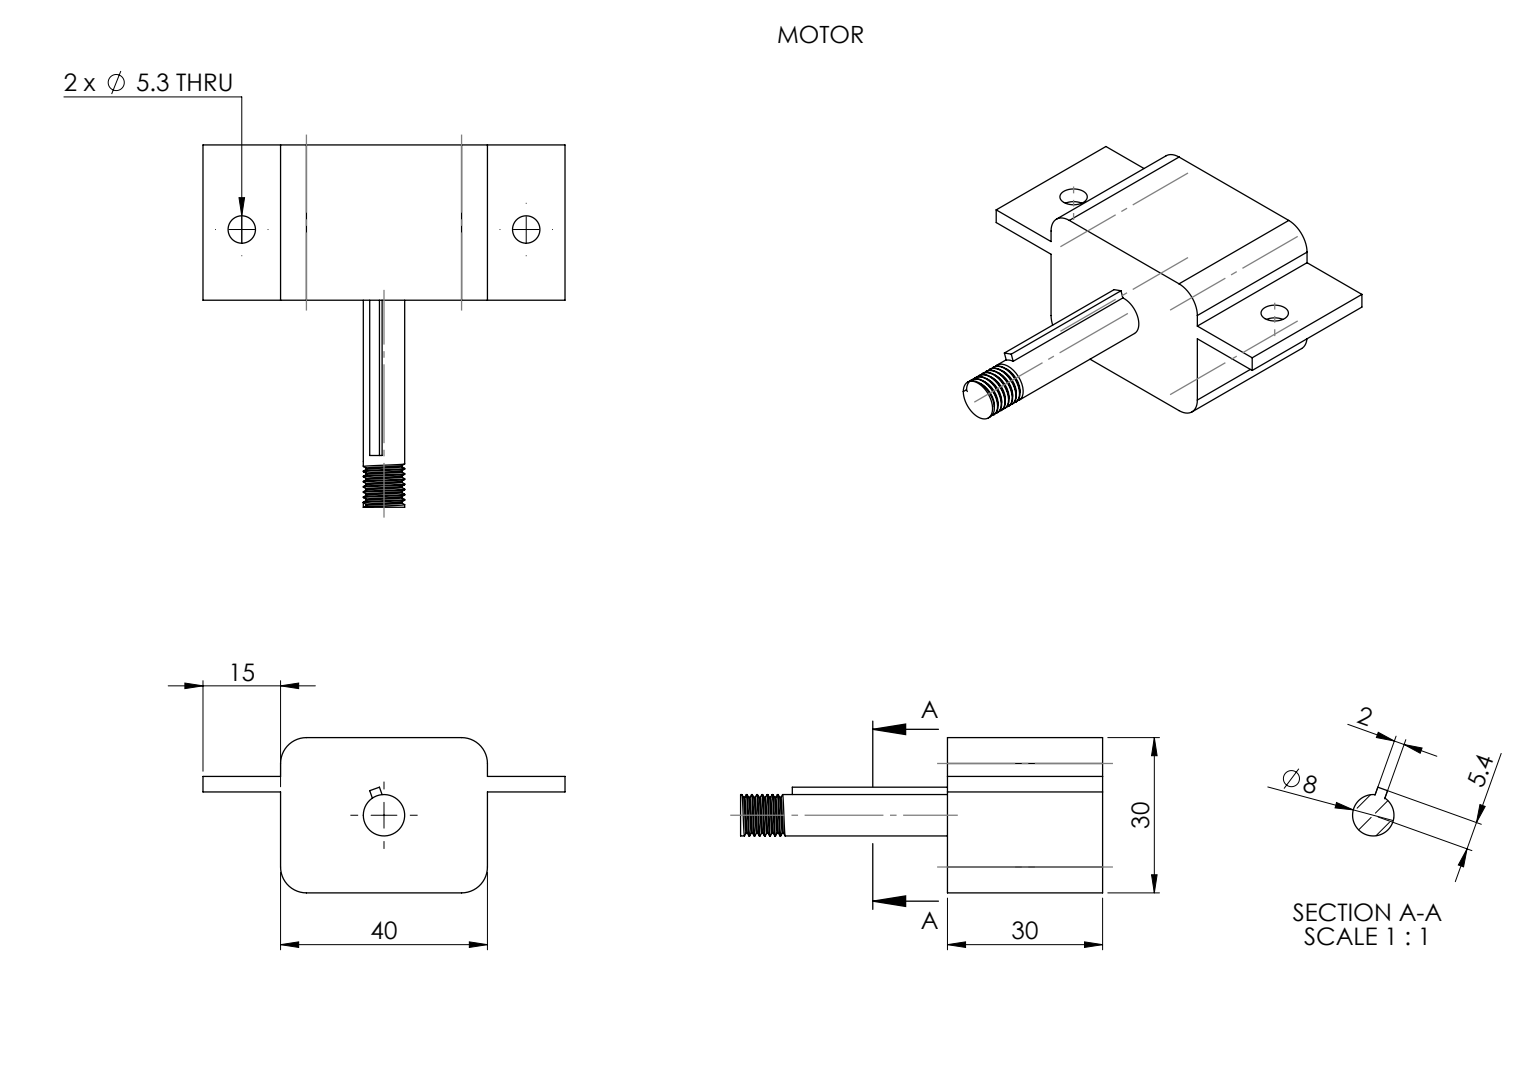
ISO-10303-21;
HEADER;
FILE_DESCRIPTION (('STEP AP214'),
    '1' );
FILE_NAME ('motor.step',
    '2026-10-08T13:46:47',
    ( '' ),
    ( '' ),
    'SwSTEP 2.0',
    'SolidWorks 2026',
    '' );
FILE_SCHEMA (( 'AUTOMOTIVE_DESIGN' ));
ENDSEC;

DATA;
#1=CARTESIAN_POINT ( 'NONE',  ( -3.999999999999999112, 1.656854249492380804, 17.93750000000000711 ) ) ;
#3=VECTOR ( 'NONE', #11246, 1000.000000000000000 ) ;
#10=DIRECTION ( 'NONE',  ( -0.000000000000000000, -0.000000000000000000, -1.000000000000000000 ) ) ;
#11=CARTESIAN_POINT ( 'NONE',  ( 1.432654583217641164, 3.458734125000000326, 19.12500000136560629 ) ) ;
#16=CARTESIAN_POINT ( 'NONE',  ( 2.445694354108821855, -2.445694354108820079, 11.81250000136560629 ) ) ;
#34=CARTESIAN_POINT ( 'NONE',  ( -1.432654583217639832, -3.458734125000000326, 12.87500000136560629 ) ) ;
#40=CARTESIAN_POINT ( 'NONE',  ( -3.999999999999999112, 0.000000000000000000, 16.12500000273119838 ) ) ;
#41=CARTESIAN_POINT ( 'NONE',  ( -20.00000000000000711, 9.999999999999964473, -19.99999999999999645 ) ) ;
#44=CYLINDRICAL_SURFACE ( 'NONE', #19665, 4.000000000000000000 ) ;
#50=ORIENTED_EDGE ( 'NONE', *, *, #19475, .F. ) ;
#51=CARTESIAN_POINT ( 'NONE',  ( -3.999999999999999112, 1.656854249492380804, 17.93750000000000711 ) ) ;
#54=ORIENTED_EDGE ( 'NONE', *, *, #9397, .T. ) ;
#64=CARTESIAN_POINT ( 'NONE',  ( -2.445694354108819191, 2.445694354108820523, 10.31250000136560629 ) ) ;
#82=ADVANCED_FACE ( 'NONE', ( #16139 ), #13987, .T. ) ;
#87=CARTESIAN_POINT ( 'NONE',  ( -2.828427124746189403, 2.828427124746190291, 10.87500000000001066 ) ) ;
#108=CARTESIAN_POINT ( 'NONE',  ( 4.000000000000000888, 4.898587196589412829E-16, 18.50000000000001066 ) ) ;
#110=EDGE_CURVE ( 'NONE', #1631, #9768, #19532, .T. ) ;
#115=ORIENTED_EDGE ( 'NONE', *, *, #19552, .T. ) ;
#121=CARTESIAN_POINT ( 'NONE',  ( 1.025207404391860050E-15, 3.458734125000000326, 19.18750000136560629 ) ) ;
#124=CARTESIAN_POINT ( 'NONE',  ( -3.999999999999999112, 0.000000000000000000, 13.00000000000001066 ) ) ;
#125=CARTESIAN_POINT ( 'NONE',  ( 1.432654583217641164, 3.458734125000000326, 12.12500000136560629 ) ) ;
#139=CARTESIAN_POINT ( 'NONE',  ( 1.025207404391860050E-15, 3.458734125000000770, 19.43750000136560629 ) ) ;
#149=DIRECTION ( 'NONE',  ( -0.000000000000000000, 1.000000000000000000, -0.000000000000000000 ) ) ;
#152=CARTESIAN_POINT ( 'NONE',  ( 2.828427124746191179, 2.828427124746190291, 16.75000000273119838 ) ) ;
#158=VERTEX_POINT ( 'NONE', #14232 ) ;
#164=CARTESIAN_POINT ( 'NONE',  ( 1.971781867644420635E-15, -4.000000000000000000, 16.25000000000001066 ) ) ;
#171=ADVANCED_FACE ( 'NONE', ( #19699 ), #12685, .T. ) ;
#180=CARTESIAN_POINT ( 'NONE',  ( 3.458734125000002546, -1.432654583217639610, 15.12500000136560807 ) ) ;
#183=CARTESIAN_POINT ( 'NONE',  ( 9.920644283265380691E-16, 4.000000000000000000, 16.75000000000001066 ) ) ;
#185=CARTESIAN_POINT ( 'NONE',  ( 1.656854249492381470, 4.000000000000000000, 11.81250000273119660 ) ) ;
#188=EDGE_LOOP ( 'NONE', ( #20058, #4346, #18980, #11606 ) ) ;
#189=ORIENTED_EDGE ( 'NONE', *, *, #1029, .F. ) ;
#190=LINE ( 'NONE', #7521, #665 ) ;
#194=CARTESIAN_POINT ( 'NONE',  ( -2.828427124746188515, -2.828427124746190735, 18.12500000000001066 ) ) ;
#202=CARTESIAN_POINT ( 'NONE',  ( 9.920644283265380691E-16, 4.000000000000000000, 15.87500000273119660 ) ) ;
#207=CARTESIAN_POINT ( 'NONE',  ( -2.762848947613220307, 4.746226468750993632, -19.99999999999999645 ) ) ;
#225=CARTESIAN_POINT ( 'NONE',  ( 4.000000000000000888, 4.898587196589412829E-16, 15.50000000000001066 ) ) ;
#234=CARTESIAN_POINT ( 'NONE',  ( 1.432654583217643163, -3.458734124999999437, 15.75000000136560629 ) ) ;
#238=CARTESIAN_POINT ( 'NONE',  ( -3.458734124999998993, 1.432654583217640276, 12.37500000136560629 ) ) ;
#251=CARTESIAN_POINT ( 'NONE',  ( 3.458734125000001658, 1.432654583217640498, 17.25000000136560629 ) ) ;
#257=CARTESIAN_POINT ( 'NONE',  ( 3.458734125000001658, 1.432654583217640498, 13.25000000136560274 ) ) ;
#263=CARTESIAN_POINT ( 'NONE',  ( -1.432654583217638944, 3.458734125000000326, 12.25000000136560629 ) ) ;
#264=CARTESIAN_POINT ( 'NONE',  ( 4.000000000000001776, -1.656854249492379694, 16.56250000273119838 ) ) ;
#265=DIRECTION ( 'NONE',  ( -1.000000000000000000, 0.000000000000000000, 0.000000000000000000 ) ) ;
#272=ORIENTED_EDGE ( 'NONE', *, *, #1937, .F. ) ;
#277=EDGE_LOOP ( 'NONE', ( #17839, #20951 ) ) ;
#278=CARTESIAN_POINT ( 'NONE',  ( 4.000000000000001776, -1.656854249492379694, 13.43750000000001243 ) ) ;
#285=DIRECTION ( 'NONE',  ( -0.000000000000000000, -0.000000000000000000, -1.000000000000000000 ) ) ;
#294=CARTESIAN_POINT ( 'NONE',  ( 1.432654583217641386, 3.458734125000000770, 13.37500000136560452 ) ) ;
#303=CARTESIAN_POINT ( 'NONE',  ( -2.247776618166699603, 3.308700692843501656, 21.31370849898476649 ) ) ;
#315=VERTEX_POINT ( 'NONE', #10985 ) ;
#323=CARTESIAN_POINT ( 'NONE',  ( 1.656854249492384135, -3.999999999999999112, 17.43750000273119483 ) ) ;
#332=ORIENTED_EDGE ( 'NONE', *, *, #12450, .T. ) ;
#343=CARTESIAN_POINT ( 'NONE',  ( 1.656854249492384135, -3.999999999999999112, 16.43750000273119838 ) ) ;
#350=CARTESIAN_POINT ( 'NONE',  ( -2.828427124746189403, 2.828427124746190291, 12.87500000000001066 ) ) ;
#355=AXIS2_PLACEMENT_3D ( 'NONE', #12842, #20101, #14526 ) ;
#361=CARTESIAN_POINT ( 'NONE',  ( 1.025207404391860050E-15, 3.458734125000000326, 17.18750000136560274 ) ) ;
#367=CARTESIAN_POINT ( 'NONE',  ( -2.445694354108819191, 2.445694354108820523, 15.31250000136560452 ) ) ;
#381=CARTESIAN_POINT ( 'NONE',  ( 1.432654583217641386, 3.458734125000000770, 15.37500000136560807 ) ) ;
#383=VECTOR ( 'NONE', #917, 1000.000000000000000 ) ;
#385=AXIS2_PLACEMENT_3D ( 'NONE', #6028, #512, #265 ) ;
#389=CARTESIAN_POINT ( 'NONE',  ( 2.445694354108822299, -2.445694354108820079, 12.06250000136560629 ) ) ;
#395=CARTESIAN_POINT ( 'NONE',  ( -3.999999999999999112, 0.000000000000000000, 17.12500000273119838 ) ) ;
#396=EDGE_CURVE ( 'NONE', #2255, #17303, #7746, .T. ) ;
#409=CARTESIAN_POINT ( 'NONE',  ( 4.000000000000001776, -1.656854249492379694, 12.43750000000001066 ) ) ;
#423=CARTESIAN_POINT ( 'NONE',  ( -1.432654583217639832, -3.458734125000000326, 14.87500000136560807 ) ) ;
#427=CARTESIAN_POINT ( 'NONE',  ( 2.828427124746191179, 2.828427124746190291, 16.62500000000001066 ) ) ;
#429=CARTESIAN_POINT ( 'NONE',  ( -2.828427124746188515, -2.828427124746190735, 14.12500000000001066 ) ) ;
#447=CARTESIAN_POINT ( 'NONE',  ( -1.656854249492380138, -3.999999999999999112, 13.31250000273119660 ) ) ;
#455=EDGE_CURVE ( 'NONE', #7307, #20911, #18012, .T. ) ;
#471=CARTESIAN_POINT ( 'NONE',  ( -2.828427124746189403, 2.828427124746190291, 13.87500000000001066 ) ) ;
#482=CARTESIAN_POINT ( 'NONE',  ( 3.458734125000001214, 1.432654583217640498, 14.00000000136560629 ) ) ;
#488=CARTESIAN_POINT ( 'NONE',  ( 2.445694354108821855, -2.445694354108820079, 13.81250000136560629 ) ) ;
#491=CARTESIAN_POINT ( 'NONE',  ( -2.828427124746189403, 2.828427124746190291, 16.00000000273119838 ) ) ;
#500=CARTESIAN_POINT ( 'NONE',  ( 1.432654583217643163, -3.458734124999999882, 15.00000000136560629 ) ) ;
#510=CARTESIAN_POINT ( 'NONE',  ( -2.445694354108819191, 2.445694354108820523, 10.31250000136560629 ) ) ;
#511=CARTESIAN_POINT ( 'NONE',  ( 1.971781867644420635E-15, -4.000000000000000000, 14.37500000273119660 ) ) ;
#512=DIRECTION ( 'NONE',  ( -1.224646799147353207E-16, 0.000000000000000000, -1.000000000000000000 ) ) ;
#514=ORIENTED_EDGE ( 'NONE', *, *, #14781, .F. ) ;
#523=CARTESIAN_POINT ( 'NONE',  ( 1.656854249492384135, -3.999999999999999112, 12.31250000000001243 ) ) ;
#536=CARTESIAN_POINT ( 'NONE',  ( -1.432654583217639166, 3.458734125000000770, 16.50000000136560629 ) ) ;
#554=CARTESIAN_POINT ( 'NONE',  ( 4.000000000000000888, 4.898587196589412829E-16, 19.50000000000001066 ) ) ;
#558=CARTESIAN_POINT ( 'NONE',  ( 2.828427124746191179, 2.828427124746190291, 13.75000000273119483 ) ) ;
#562=CARTESIAN_POINT ( 'NONE',  ( 3.458734125000001214, 1.432654583217640498, 19.00000000136560629 ) ) ;
#582=CARTESIAN_POINT ( 'NONE',  ( 4.000000000000000888, 4.898587196589412829E-16, 13.50000000000001066 ) ) ;
#587=CARTESIAN_POINT ( 'NONE',  ( 27.50000000000000000, 4.500000000000001776, -36.31025403784445871 ) ) ;
#590=VECTOR ( 'NONE', #2193, 1000.000000000000000 ) ;
#594=CARTESIAN_POINT ( 'NONE',  ( 1.432654583217641164, 3.458734125000000326, 13.12500000136560274 ) ) ;
#598=CARTESIAN_POINT ( 'NONE',  ( -3.999999999999999112, 1.656854249492380582, 12.93750000000001066 ) ) ;
#613=ORIENTED_EDGE ( 'NONE', *, *, #10738, .T. ) ;
#614=CARTESIAN_POINT ( 'NONE',  ( 1.025207404391860050E-15, 3.458734125000000770, 18.43750000136560629 ) ) ;
#625=CARTESIAN_POINT ( 'NONE',  ( 2.445694354108821855, -2.445694354108820079, 10.81250000136560452 ) ) ;
#626=CARTESIAN_POINT ( 'NONE',  ( 2.828427124746191179, 2.828427124746190291, 11.75000000273119660 ) ) ;
#629=ORIENTED_EDGE ( 'NONE', *, *, #21485, .F. ) ;
#634=CARTESIAN_POINT ( 'NONE',  ( 2.828427124746192067, -2.828427124746189847, 11.37500000000001066 ) ) ;
#636=EDGE_CURVE ( 'NONE', #21119, #17601, #4711, .T. ) ;
#644=CARTESIAN_POINT ( 'NONE',  ( -3.458734124999998105, -1.432654583217642497, 18.75000000136560985 ) ) ;
#645=CARTESIAN_POINT ( 'NONE',  ( 4.000000000000000888, 4.898587196589412829E-16, 11.50000000000001066 ) ) ;
#651=CARTESIAN_POINT ( 'NONE',  ( -1.432654583217639166, 3.458734125000000770, 14.50000000136560629 ) ) ;
#652=DIRECTION ( 'NONE',  ( -1.224646799147353207E-16, 0.000000000000000000, -1.000000000000000000 ) ) ;
#659=ORIENTED_EDGE ( 'NONE', *, *, #9537, .F. ) ;
#662=CARTESIAN_POINT ( 'NONE',  ( 4.000000000000000888, 4.898587196589412829E-16, 21.31370849898476649 ) ) ;
#665=VECTOR ( 'NONE', #22333, 1000.000000000000000 ) ;
#673=( BOUNDED_CURVE ( )  B_SPLINE_CURVE ( 2, ( #7283, #9203, #16490, #14354, #12440, #10774, #7037, #12692, #3655 ),
 .UNSPECIFIED., .F., .F. ) 
 B_SPLINE_CURVE_WITH_KNOTS ( ( 3, 2, 2, 2, 3 ),
 ( 0.05000000000000000278, 0.06250000000000000000, 0.07499999999999999722, 0.08749999999999999445, 0.1000000000000000056 ),
 .UNSPECIFIED. ) 
 CURVE ( )  GEOMETRIC_REPRESENTATION_ITEM ( )  RATIONAL_B_SPLINE_CURVE ( ( 1.000000000000000000, 0.9238795325112867385, 1.000000000000000000, 0.9238795325112867385, 1.000000000000000000, 0.9238795325112867385, 1.000000000000000000, 0.9238795325112867385, 1.000000000000000000 ) ) 
 REPRESENTATION_ITEM ( '' )  );
#676=CARTESIAN_POINT ( 'NONE',  ( -2.445694354108818303, -2.445694354108820523, 18.56250000136560629 ) ) ;
#694=FACE_OUTER_BOUND ( 'NONE', #17938, .T. ) ;
#698=CARTESIAN_POINT ( 'NONE',  ( 4.000000000000000888, 1.656854249492381248, 16.56250000000001066 ) ) ;
#706=ADVANCED_FACE ( 'NONE', ( #20086 ), #19862, .T. ) ;
#709=DIRECTION ( 'NONE',  ( -0.000000000000000000, -0.000000000000000000, -1.000000000000000000 ) ) ;
#712=CARTESIAN_POINT ( 'NONE',  ( 2.445694354108821855, -2.445694354108820079, 11.81250000136560629 ) ) ;
#724=ORIENTED_EDGE ( 'NONE', *, *, #7005, .T. ) ;
#725=CARTESIAN_POINT ( 'NONE',  ( -3.999999999999999112, 0.000000000000000000, 16.12500000273119838 ) ) ;
#736=CARTESIAN_POINT ( 'NONE',  ( -2.445694354108818303, -2.445694354108820967, 16.81250000136560629 ) ) ;
#749=CARTESIAN_POINT ( 'NONE',  ( -3.999999999999998224, -1.656854249492383246, 13.18750000273119660 ) ) ;
#756=CARTESIAN_POINT ( 'NONE',  ( -2.828427124746189403, 2.828427124746190291, 17.00000000273119838 ) ) ;
#764=CARTESIAN_POINT ( 'NONE',  ( 1.656854249492384135, -3.999999999999999112, 14.31250000000001066 ) ) ;
#767=ORIENTED_EDGE ( 'NONE', *, *, #14910, .F. ) ;
#772=CARTESIAN_POINT ( 'NONE',  ( 2.445694354108822299, -2.445694354108820079, 18.06250000136560274 ) ) ;
#774=VECTOR ( 'NONE', #12841, 1000.000000000000000 ) ;
#780=CARTESIAN_POINT ( 'NONE',  ( 3.458734125000001658, 1.432654583217640498, 12.25000000136560452 ) ) ;
#781=ADVANCED_FACE ( 'NONE', ( #23460 ), #8880, .F. ) ;
#784=EDGE_CURVE ( 'NONE', #20532, #22990, #16520, .T. ) ;
#786=LINE ( 'NONE', #11832, #6692 ) ;
#795=EDGE_LOOP ( 'NONE', ( #3413, #2892, #4216, #3819, #4414, #8132, #9324, #7494, #20640, #8419, #9699, #7965, #332, #11494, #6870, #4116, #6329, #19356, #12885, #18929, #9383, #2214 ) ) ;
#800=ORIENTED_EDGE ( 'NONE', *, *, #8131, .T. ) ;
#801=FACE_OUTER_BOUND ( 'NONE', #1222, .T. ) ;
#803=CARTESIAN_POINT ( 'NONE',  ( -1.432654583217638944, 3.458734125000000326, 18.25000000136560629 ) ) ;
#819=ADVANCED_FACE ( 'NONE', ( #14739 ), #5612, .T. ) ;
#821=CARTESIAN_POINT ( 'NONE',  ( 4.000000000000000888, 1.656854249492381248, 12.56250000000001243 ) ) ;
#823=CARTESIAN_POINT ( 'NONE',  ( 4.000000000000000888, 4.898587196589412829E-16, 19.50000000000001066 ) ) ;
#824=( BOUNDED_CURVE ( )  B_SPLINE_CURVE ( 2, ( #13954, #15639, #17660, #1221, #6398, #22911, #21329, #10248, #6525 ),
 .UNSPECIFIED., .F., .F. ) 
 B_SPLINE_CURVE_WITH_KNOTS ( ( 3, 2, 2, 2, 3 ),
 ( 0.000000000000000000, 0.01250000000000000243, 0.02500000000000000486, 0.03749999999999999861, 0.05000000000000000971 ),
 .UNSPECIFIED. ) 
 CURVE ( )  GEOMETRIC_REPRESENTATION_ITEM ( )  RATIONAL_B_SPLINE_CURVE ( ( 1.000000000000000000, 0.9238795325112867385, 1.000000000000000000, 0.9238795325112867385, 1.000000000000000000, 0.9238795325112867385, 1.000000000000000000, 0.9238795325112867385, 1.000000000000000000 ) ) 
 REPRESENTATION_ITEM ( '' )  );
#830=CARTESIAN_POINT ( 'NONE',  ( 1.872352939448454495E-15, -3.458734125000000326, 11.68750000136560629 ) ) ;
#832=CYLINDRICAL_SURFACE ( 'NONE', #7334, 4.999999999999997335 ) ;
#836=CARTESIAN_POINT ( 'NONE',  ( 1.872352939448454495E-15, -3.458734125000000326, 10.68750000136560452 ) ) ;
#839=VERTEX_POINT ( 'NONE', #9344 ) ;
#848=CARTESIAN_POINT ( 'NONE',  ( -2.445694354108818303, -2.445694354108820967, 13.81250000136560629 ) ) ;
#856=PLANE ( 'NONE',  #19991 ) ;
#859=CARTESIAN_POINT ( 'NONE',  ( -3.999999999999999112, 0.000000000000000000, 10.12500000273119660 ) ) ;
#860=FACE_OUTER_BOUND ( 'NONE', #12699, .T. ) ;
#863=EDGE_LOOP ( 'NONE', ( #11160, #1862, #19901, #14870 ) ) ;
#867=ORIENTED_EDGE ( 'NONE', *, *, #22089, .F. ) ;
#878=DIRECTION ( 'NONE',  ( -0.000000000000000000, -0.000000000000000000, -1.000000000000000000 ) ) ;
#891=DIRECTION ( 'NONE',  ( -1.224646799147353207E-16, 0.000000000000000000, -1.000000000000000000 ) ) ;
#893=CARTESIAN_POINT ( 'NONE',  ( -3.999999999999999112, 0.000000000000000000, 14.00000000000001066 ) ) ;
#913=CARTESIAN_POINT ( 'NONE',  ( 1.872352939448454495E-15, -3.458734125000000326, 18.68750000136560629 ) ) ;
#916=ORIENTED_EDGE ( 'NONE', *, *, #11727, .T. ) ;
#917=DIRECTION ( 'NONE',  ( -0.000000000000000000, -0.000000000000000000, -1.000000000000000000 ) ) ;
#927=CYLINDRICAL_SURFACE ( 'NONE', #10317, 4.000000000000000000 ) ;
#940=CARTESIAN_POINT ( 'NONE',  ( -3.458734124999998993, 1.432654583217640276, 14.37500000136560452 ) ) ;
#950=CARTESIAN_POINT ( 'NONE',  ( 1.025207404391860050E-15, 3.458734125000000326, 10.18750000136560629 ) ) ;
#953=DIRECTION ( 'NONE',  ( 0.000000000000000000, 0.000000000000000000, 1.000000000000000000 ) ) ;
#961=CARTESIAN_POINT ( 'NONE',  ( 3.458734125000001658, 4.235727675282972223E-16, 13.18750000136560452 ) ) ;
#976=CARTESIAN_POINT ( 'NONE',  ( 1.656854249492384135, -3.999999999999999112, 13.43750000273119838 ) ) ;
#977=DIRECTION ( 'NONE',  ( 0.3373062947069098150, -0.9413949561959078505, 0.000000000000000000 ) ) ;
#988=DIRECTION ( 'NONE',  ( 1.000000000000000000, 0.000000000000000000, 0.000000000000000000 ) ) ;
#996=DIRECTION ( 'NONE',  ( -0.000000000000000000, -0.000000000000000000, -1.000000000000000000 ) ) ;
#998=CARTESIAN_POINT ( 'NONE',  ( 2.828427124746191179, 2.828427124746190291, 15.75000000273119660 ) ) ;
#1006=CARTESIAN_POINT ( 'NONE',  ( 1.432654583217643163, -3.458734124999999882, 13.00000000136560629 ) ) ;
#1012=CARTESIAN_POINT ( 'NONE',  ( 4.000000000000000888, 4.898587196589412829E-16, 15.62500000273119660 ) ) ;
#1013=PRESENTATION_STYLE_ASSIGNMENT (( #17448 ) ) ;
#1029=EDGE_CURVE ( 'NONE', #4019, #13418, #23047, .T. ) ;
#1031=CARTESIAN_POINT ( 'NONE',  ( -2.445694354108819191, 2.445694354108820523, 19.31250000136560629 ) ) ;
#1049=CARTESIAN_POINT ( 'NONE',  ( 2.828427124746191179, 2.828427124746190291, 17.62500000000001066 ) ) ;
#1053=CARTESIAN_POINT ( 'NONE',  ( -3.999999999999999112, 0.000000000000000000, 12.00000000000001066 ) ) ;
#1060=CARTESIAN_POINT ( 'NONE',  ( -1.432654583217639166, 3.458734125000000770, 18.50000000136560629 ) ) ;
#1065=CARTESIAN_POINT ( 'NONE',  ( 1.656854249492381470, 4.000000000000000000, 15.68750000000001066 ) ) ;
#1080=CARTESIAN_POINT ( 'NONE',  ( -3.458734124999999437, 1.432654583217640498, 11.62500000136560452 ) ) ;
#1092=CARTESIAN_POINT ( 'NONE',  ( 4.000000000000000888, 4.898587196589412829E-16, 12.62500000273119660 ) ) ;
#1112=CARTESIAN_POINT ( 'NONE',  ( -3.458734124999998105, -1.432654583217642497, 17.75000000136560274 ) ) ;
#1113=CARTESIAN_POINT ( 'NONE',  ( -2.828427124746188515, -2.828427124746190735, 14.25000000273119660 ) ) ;
#1114=VECTOR ( 'NONE', #23199, 1000.000000000000000 ) ;
#1127=CARTESIAN_POINT ( 'NONE',  ( 1.971781867644420635E-15, -4.000000000000000000, 15.37500000273119660 ) ) ;
#1128=( NAMED_UNIT ( * ) PLANE_ANGLE_UNIT ( ) SI_UNIT ( $, .RADIAN. ) );
#1132=VERTEX_POINT ( 'NONE', #18132 ) ;
#1136=FACE_OUTER_BOUND ( 'NONE', #3145, .T. ) ;
#1138=UNCERTAINTY_MEASURE_WITH_UNIT (LENGTH_MEASURE( 1.000000000000000082E-05 ), #18255, 'distance_accuracy_value', 'NONE');
#1146=DIRECTION ( 'NONE',  ( -1.000000000000000000, 0.000000000000000000, 0.000000000000000000 ) ) ;
#1150=CARTESIAN_POINT ( 'NONE',  ( 2.445694354108821411, 2.445694354108820523, 16.06250000136560629 ) ) ;
#1166=ORIENTED_EDGE ( 'NONE', *, *, #12523, .F. ) ;
#1167=CARTESIAN_POINT ( 'NONE',  ( -3.999999999999999112, 0.000000000000000000, 20.00000000000001066 ) ) ;
#1170=CARTESIAN_POINT ( 'NONE',  ( -1.656854249492380138, -3.999999999999999112, 19.18750000000001066 ) ) ;
#1176=EDGE_CURVE ( 'NONE', #158, #17446, #12413, .T. ) ;
#1178=CARTESIAN_POINT ( 'NONE',  ( -15.00000000000001066, 10.00000000000000000, -49.99999999999999289 ) ) ;
#1181=CARTESIAN_POINT ( 'NONE',  ( 2.445694354108821855, -2.445694354108820079, 10.81250000136560452 ) ) ;
#1196=ORIENTED_EDGE ( 'NONE', *, *, #6597, .F. ) ;
#1197=CARTESIAN_POINT ( 'NONE',  ( -1.432654583217639166, 3.458734125000000770, 13.50000000136560452 ) ) ;
#1209=CARTESIAN_POINT ( 'NONE',  ( -3.458734124999998993, -1.432654583217642497, 18.50000000136560629 ) ) ;
#1221=CARTESIAN_POINT ( 'NONE',  ( -1.656854249492379472, 4.000000000000000000, 19.81250000000001776 ) ) ;
#1222=EDGE_LOOP ( 'NONE', ( #3301, #17935, #17506, #2754 ) ) ;
#1227=CARTESIAN_POINT ( 'NONE',  ( 3.458734125000001658, 1.432654583217640498, 14.25000000136560452 ) ) ;
#1228=CARTESIAN_POINT ( 'NONE',  ( -1.656854249492379250, 4.000000000000000000, 14.93750000273119660 ) ) ;
#1233=CARTESIAN_POINT ( 'NONE',  ( -3.458734124999999437, 1.432654583217640498, 11.62500000136560452 ) ) ;
#1236=EDGE_CURVE ( 'NONE', #10607, #14136, #2968, .T. ) ;
#1242=SURFACE_STYLE_FILL_AREA ( #17329 ) ;
#1256=DIRECTION ( 'NONE',  ( 1.224646799147353207E-16, -0.000000000000000000, 1.000000000000000000 ) ) ;
#1259=CARTESIAN_POINT ( 'NONE',  ( -1.432654583217638944, 3.458734125000000326, 14.25000000136560452 ) ) ;
#1270=CARTESIAN_POINT ( 'NONE',  ( 4.000000000000000888, 4.898587196589412829E-16, 13.62500000273119660 ) ) ;
#1280=DIRECTION ( 'NONE',  ( -1.224646799147353207E-16, 0.000000000000000000, -1.000000000000000000 ) ) ;
#1281=DIRECTION ( 'NONE',  ( 1.224646799147353207E-16, -0.000000000000000000, 1.000000000000000000 ) ) ;
#1288=CARTESIAN_POINT ( 'NONE',  ( 3.458734125000001214, 4.235727675282971730E-16, 10.93750000136560452 ) ) ;
#1293=DIRECTION ( 'NONE',  ( -0.000000000000000000, -1.000000000000000000, 0.000000000000000000 ) ) ;
#1309=CARTESIAN_POINT ( 'NONE',  ( 1.872352939448454495E-15, -3.458734125000000770, 11.93750000136560629 ) ) ;
#1318=DIRECTION ( 'NONE',  ( -0.000000000000000000, -0.000000000000000000, -1.000000000000000000 ) ) ;
#1323=CARTESIAN_POINT ( 'NONE',  ( 3.458734125000002102, -1.432654583217639610, 17.87500000136560274 ) ) ;
#1332=DIRECTION ( 'NONE',  ( -0.000000000000000000, -1.000000000000000000, 0.000000000000000000 ) ) ;
#1334=CYLINDRICAL_SURFACE ( 'NONE', #17915, 4.999999999999999112 ) ;
#1346=CARTESIAN_POINT ( 'NONE',  ( -2.445694354108818303, -2.445694354108820967, 15.81250000136560629 ) ) ;
#1347=CARTESIAN_POINT ( 'NONE',  ( 1.971781867644420635E-15, -4.000000000000000000, 11.37500000273119660 ) ) ;
#1362=ADVANCED_FACE ( 'NONE', ( #1828 ), #9179, .T. ) ;
#1369=DIRECTION ( 'NONE',  ( -1.000000000000000000, 0.000000000000000000, 0.000000000000000000 ) ) ;
#1377=CARTESIAN_POINT ( 'NONE',  ( 1.432654583217643163, -3.458734124999999437, 15.75000000136560629 ) ) ;
#1384=VERTEX_POINT ( 'NONE', #17980 ) ;
#1404=CARTESIAN_POINT ( 'NONE',  ( -2.445694354108818303, -2.445694354108820967, 17.81250000136560274 ) ) ;
#1409=DIRECTION ( 'NONE',  ( 0.000000000000000000, 0.000000000000000000, -1.000000000000000000 ) ) ;
#1418=EDGE_LOOP ( 'NONE', ( #4713, #10059, #19395, #21066 ) ) ;
#1423=CARTESIAN_POINT ( 'NONE',  ( -2.828427124746188515, -2.828427124746190735, 19.12500000000001066 ) ) ;
#1438=( BOUNDED_CURVE ( )  B_SPLINE_CURVE ( 2, ( #21050, #14260, #7310, #1530, #19966 ),
 .UNSPECIFIED., .F., .F. ) 
 B_SPLINE_CURVE_WITH_KNOTS ( ( 3, 2, 3 ),
 ( 0.9000000000000000222, 0.9124999999999999778, 0.9155333511103322941 ),
 .UNSPECIFIED. ) 
 CURVE ( )  GEOMETRIC_REPRESENTATION_ITEM ( )  RATIONAL_B_SPLINE_CURVE ( ( 1.000000000000000000, 0.9238795325112867385, 1.000000000000000000, 0.9815279916339278987, 0.9720211172018224932 ) ) 
 REPRESENTATION_ITEM ( '' )  );
#1442=CARTESIAN_POINT ( 'NONE',  ( -1.432654583217638944, 3.458734125000000326, 17.25000000136560274 ) ) ;
#1465=CIRCLE ( 'NONE', #16418, 2.649999999999992806 ) ;
#1466=CARTESIAN_POINT ( 'NONE',  ( 1.432654583217641386, 3.458734125000000770, 15.37500000136560807 ) ) ;
#1487=CARTESIAN_POINT ( 'NONE',  ( -2.828427124746188515, -2.828427124746190735, 19.12500000000001066 ) ) ;
#1491=AXIS2_PLACEMENT_3D ( 'NONE', #19343, #17798, #1369 ) ;
#1494=CARTESIAN_POINT ( 'NONE',  ( -15.00000000000000711, 10.00000000000000000, -19.99999999999999645 ) ) ;
#1496=CARTESIAN_POINT ( 'NONE',  ( -2.828427124746188515, -2.828427124746190735, 11.12500000000001066 ) ) ;
#1500=CIRCLE ( 'NONE', #7252, 4.999999999999997335 ) ;
#1503=CARTESIAN_POINT ( 'NONE',  ( 1.236993788156008760E-15, 0.000000000000000000, 21.31370849898476649 ) ) ;
#1505=DIRECTION ( 'NONE',  ( 1.224646799147353207E-16, -0.000000000000000000, 1.000000000000000000 ) ) ;
#1509=CARTESIAN_POINT ( 'NONE',  ( -1.432654583217638944, 3.458734125000000326, 15.25000000136560807 ) ) ;
#1511=DIRECTION ( 'NONE',  ( -1.000000000000000000, 0.000000000000000000, 0.000000000000000000 ) ) ;
#1516=ORIENTED_EDGE ( 'NONE', *, *, #9390, .T. ) ;
#1518=CARTESIAN_POINT ( 'NONE',  ( 2.828427124746191179, 2.828427124746190291, 13.75000000273119483 ) ) ;
#1527=DIRECTION ( 'NONE',  ( -1.000000000000000000, -6.123233995736827666E-17, 0.000000000000000000 ) ) ;
#1530=CARTESIAN_POINT ( 'NONE',  ( -2.560821871666743910, 3.096032377825634896, 9.985724042037038117 ) ) ;
#1534=CARTESIAN_POINT ( 'NONE',  ( -3.458734124999998993, 0.000000000000000000, 10.43750000136560452 ) ) ;
#1541=CARTESIAN_POINT ( 'NONE',  ( 1.656854249492381470, 4.000000000000000000, 10.81250000273119660 ) ) ;
#1551=CARTESIAN_POINT ( 'NONE',  ( -3.999999999999999112, 1.656854249492380582, 18.93750000000001066 ) ) ;
#1552=CARTESIAN_POINT ( 'NONE',  ( 9.920644283265380691E-16, 4.000000000000000000, 18.75000000000001066 ) ) ;
#1566=CARTESIAN_POINT ( 'NONE',  ( 1.025207404391860050E-15, 3.458734125000000326, 18.18750000136560274 ) ) ;
#1587=( BOUNDED_CURVE ( )  B_SPLINE_CURVE ( 2, ( #22498, #7559, #22375, #11170, #13439, #18441, #9361, #18802, #14881 ),
 .UNSPECIFIED., .F., .F. ) 
 B_SPLINE_CURVE_WITH_KNOTS ( ( 3, 2, 2, 2, 3 ),
 ( 0.1000000000000000056, 0.1125000000000000028, 0.1250000000000000000, 0.1375000000000000111, 0.1499999999999999944 ),
 .UNSPECIFIED. ) 
 CURVE ( )  GEOMETRIC_REPRESENTATION_ITEM ( )  RATIONAL_B_SPLINE_CURVE ( ( 1.000000000000000000, 0.9238795325112867385, 1.000000000000000000, 0.9238795325112867385, 1.000000000000000000, 0.9238795325112867385, 1.000000000000000000, 0.9238795325112867385, 1.000000000000000000 ) ) 
 REPRESENTATION_ITEM ( '' )  );
#1588=CARTESIAN_POINT ( 'NONE',  ( 3.458734125000001658, 1.432654583217640498, 16.25000000136560629 ) ) ;
#1597=VERTEX_POINT ( 'NONE', #3516 ) ;
#1606=CARTESIAN_POINT ( 'NONE',  ( -1.656854249492380138, -3.999999999999999112, 17.18750000000001066 ) ) ;
#1613=CARTESIAN_POINT ( 'NONE',  ( -2.828427124746189403, 2.828427124746190291, 11.87500000000001066 ) ) ;
#1624=CARTESIAN_POINT ( 'NONE',  ( -3.458734124999998993, 0.000000000000000000, 14.43750000136560452 ) ) ;
#1631=VERTEX_POINT ( 'NONE', #19559 ) ;
#1648=CARTESIAN_POINT ( 'NONE',  ( -2.828427124746189403, 2.828427124746190291, 16.00000000273119838 ) ) ;
#1656=DIRECTION ( 'NONE',  ( -0.000000000000000000, -0.000000000000000000, -1.000000000000000000 ) ) ;
#1664=DIRECTION ( 'NONE',  ( -0.000000000000000000, -0.000000000000000000, -1.000000000000000000 ) ) ;
#1671=CARTESIAN_POINT ( 'NONE',  ( 1.971781867644420635E-15, -4.000000000000000000, 19.25000000000001066 ) ) ;
#1678=FACE_OUTER_BOUND ( 'NONE', #863, .T. ) ;
#1683=CARTESIAN_POINT ( 'NONE',  ( 1.025207404391860050E-15, 3.458734125000000326, 16.18750000136560629 ) ) ;
#1699=ADVANCED_FACE ( 'NONE', ( #3394 ), #12407, .F. ) ;
#1701=CARTESIAN_POINT ( 'NONE',  ( 2.445694354108821411, 2.445694354108820523, 14.31250000136560452 ) ) ;
#1720=CARTESIAN_POINT ( 'NONE',  ( 2.828427124746192067, -2.828427124746189847, 18.37500000000001066 ) ) ;
#1749=CARTESIAN_POINT ( 'NONE',  ( 34.99999999999999289, 4.500000000000001776, -50.00000000000000000 ) ) ;
#1762=LINE ( 'NONE', #19728, #17185 ) ;
#1764=CARTESIAN_POINT ( 'NONE',  ( -2.828427124746188515, -2.828427124746190735, 17.25000000273119838 ) ) ;
#1770=EDGE_CURVE ( 'NONE', #13418, #16438, #7330, .T. ) ;
#1776=ORIENTED_EDGE ( 'NONE', *, *, #5722, .F. ) ;
#1781=DIRECTION ( 'NONE',  ( 0.000000000000000000, 0.000000000000000000, 1.000000000000000000 ) ) ;
#1782=ORIENTED_EDGE ( 'NONE', *, *, #14781, .T. ) ;
#1784=CARTESIAN_POINT ( 'NONE',  ( -3.999999999999999112, 0.000000000000000000, 21.31370849898476649 ) ) ;
#1785=CARTESIAN_POINT ( 'NONE',  ( -2.828427124746188515, -2.828427124746190735, 18.12500000000001066 ) ) ;
#1790=VECTOR ( 'NONE', #4055, 1000.000000000000000 ) ;
#1791=AXIS2_PLACEMENT_3D ( 'NONE', #12896, #285, #12679 ) ;
#1795=CARTESIAN_POINT ( 'NONE',  ( 3.458734125000002102, -1.432654583217639610, 18.87500000136560274 ) ) ;
#1798=CARTESIAN_POINT ( 'NONE',  ( -0.3649867057748643617, 3.983313282257324950, 10.00000000000000888 ) ) ;
#1799=CARTESIAN_POINT ( 'NONE',  ( 1.872352939448454495E-15, -3.458734125000000326, 12.68750000136560629 ) ) ;
#1809=CARTESIAN_POINT ( 'NONE',  ( 1.656854249492384135, -3.999999999999999112, 17.31250000000001066 ) ) ;
#1818=CARTESIAN_POINT ( 'NONE',  ( 1.872352939448454495E-15, -3.458734125000000770, 10.93750000136560452 ) ) ;
#1819=CARTESIAN_POINT ( 'NONE',  ( 1.656854249492384135, -3.999999999999999112, 10.43750000273119660 ) ) ;
#1825=FACE_OUTER_BOUND ( 'NONE', #22054, .T. ) ;
#1826=LINE ( 'NONE', #21939, #17225 ) ;
#1828=FACE_OUTER_BOUND ( 'NONE', #2269, .T. ) ;
#1830=EDGE_LOOP ( 'NONE', ( #514, #19043, #17039, #9791 ) ) ;
#1836=CARTESIAN_POINT ( 'NONE',  ( -3.999999999999999112, 0.000000000000000000, 16.00000000000001066 ) ) ;
#1857=DIRECTION ( 'NONE',  ( 0.000000000000000000, 0.000000000000000000, 1.000000000000000000 ) ) ;
#1862=ORIENTED_EDGE ( 'NONE', *, *, #14206, .T. ) ;
#1876=STYLED_ITEM ( 'NONE', ( #1013 ), #19027 ) ;
#1881=CARTESIAN_POINT ( 'NONE',  ( -3.999999999999999112, 0.000000000000000000, 11.00000000000001066 ) ) ;
#1882=CARTESIAN_POINT ( 'NONE',  ( 1.236993788156008760E-15, 0.000000000000000000, -20.00000000000000000 ) ) ;
#1894=EDGE_CURVE ( 'NONE', #18318, #20532, #21936, .T. ) ;
#1906=CARTESIAN_POINT ( 'NONE',  ( 2.828427124746192067, -2.828427124746189847, 19.37500000000001066 ) ) ;
#1911=CYLINDRICAL_SURFACE ( 'NONE', #355, 2.649999999999992806 ) ;
#1918=CARTESIAN_POINT ( 'NONE',  ( 3.458734125000001214, 4.235727675282971730E-16, 15.93750000136560629 ) ) ;
#1922=CARTESIAN_POINT ( 'NONE',  ( -2.445694354108818303, -2.445694354108820523, 12.56250000136560629 ) ) ;
#1934=CARTESIAN_POINT ( 'NONE',  ( -3.458734124999999437, 0.000000000000000000, 19.68750000136560629 ) ) ;
#1937=EDGE_CURVE ( 'NONE', #21119, #4764, #20733, .T. ) ;
#1941=CARTESIAN_POINT ( 'NONE',  ( -2.445694354108819191, 2.445694354108820523, 12.56250000136560629 ) ) ;
#1947=CARTESIAN_POINT ( 'NONE',  ( -3.999999999999999112, 1.656854249492380804, 16.06250000273119838 ) ) ;
#1958=CARTESIAN_POINT ( 'NONE',  ( 2.828427124746192067, -2.828427124746189847, 16.37500000000001066 ) ) ;
#1970=CARTESIAN_POINT ( 'NONE',  ( -3.458734124999999437, 1.432654583217640498, 15.62500000136560629 ) ) ;
#1975=CARTESIAN_POINT ( 'NONE',  ( -3.999999999999999112, 0.000000000000000000, 12.12500000273119838 ) ) ;
#1991=CARTESIAN_POINT ( 'NONE',  ( -3.999999999999999112, 1.656854249492380804, 10.93750000000001421 ) ) ;
#2000=ORIENTED_EDGE ( 'NONE', *, *, #1770, .T. ) ;
#2010=CARTESIAN_POINT ( 'NONE',  ( -3.999999999999999112, 0.000000000000000000, 10.12500000273119660 ) ) ;
#2014=CARTESIAN_POINT ( 'NONE',  ( -1.656854249492379472, 4.000000000000000000, 18.93750000273119838 ) ) ;
#2015=CARTESIAN_POINT ( 'NONE',  ( 4.000000000000000888, 4.898587196589412829E-16, 14.50000000000001066 ) ) ;
#2016=CARTESIAN_POINT ( 'NONE',  ( -14.99999999999997335, -15.00000000000000000, -49.99999999999999289 ) ) ;
#2022=ADVANCED_FACE ( 'NONE', ( #21083, #15623 ), #856, .T. ) ;
#2028=CARTESIAN_POINT ( 'NONE',  ( -2.445694354108819191, 2.445694354108820523, 16.31250000136560629 ) ) ;
#2029=DIRECTION ( 'NONE',  ( 1.224646799147353207E-16, 0.000000000000000000, 1.000000000000000000 ) ) ;
#2033=CARTESIAN_POINT ( 'NONE',  ( 2.445694354108821411, 2.445694354108820523, 12.06250000136560629 ) ) ;
#2050=CARTESIAN_POINT ( 'NONE',  ( -3.458734124999998105, -1.432654583217642497, 10.75000000136560452 ) ) ;
#2057=CARTESIAN_POINT ( 'NONE',  ( -3.458734124999998105, -1.432654583217642275, 12.50000000136560629 ) ) ;
#2058=CARTESIAN_POINT ( 'NONE',  ( 4.000000000000000888, 4.898587196589412829E-16, 15.62500000273119660 ) ) ;
#2062=ORIENTED_EDGE ( 'NONE', *, *, #3302, .F. ) ;
#2071=CARTESIAN_POINT ( 'NONE',  ( 4.000000000000000888, 4.898587196589412829E-16, 13.50000000000001066 ) ) ;
#2073=VECTOR ( 'NONE', #10600, 1000.000000000000114 ) ;
#2077=DIRECTION ( 'NONE',  ( 0.000000000000000000, -1.000000000000000000, 0.000000000000000000 ) ) ;
#2087=CARTESIAN_POINT ( 'NONE',  ( -1.432654583217639166, 3.458734125000000770, 13.50000000136560452 ) ) ;
#2102=EDGE_LOOP ( 'NONE', ( #18696, #19564, #15462, #18201, #5418 ) ) ;
#2110=CARTESIAN_POINT ( 'NONE',  ( -1.656854249492379250, 4.000000000000000000, 18.93750000273119838 ) ) ;
#2117=CARTESIAN_POINT ( 'NONE',  ( -27.50000000000000711, 4.500000000000001776, -36.31025403784445871 ) ) ;
#2122=CARTESIAN_POINT ( 'NONE',  ( 2.828427124746192067, -2.828427124746189847, 12.37500000000001066 ) ) ;
#2130=CARTESIAN_POINT ( 'NONE',  ( -2.828427124746188515, -2.828427124746190735, 16.25000000273119838 ) ) ;
#2134=EDGE_CURVE ( 'NONE', #22281, #13130, #10470, .T. ) ;
#2136=CARTESIAN_POINT ( 'NONE',  ( -2.828427124746189403, 2.828427124746190291, 15.87500000000001066 ) ) ;
#2144=CARTESIAN_POINT ( 'NONE',  ( 1.236993788156008760E-15, 0.000000000000000000, 21.31370849898476649 ) ) ;
#2146=CARTESIAN_POINT ( 'NONE',  ( -3.458734124999998993, 0.000000000000000000, 17.43750000136560274 ) ) ;
#2147=CARTESIAN_POINT ( 'NONE',  ( 19.99999999999998934, 7.500000000000001776, -50.00000000000000000 ) ) ;
#2151=CARTESIAN_POINT ( 'NONE',  ( -1.432654583217639610, -3.458734124999999882, 14.62500000136560629 ) ) ;
#2152=DIRECTION ( 'NONE',  ( -0.000000000000000000, -0.000000000000000000, -1.000000000000000000 ) ) ;
#2162=ADVANCED_FACE ( 'NONE', ( #1678 ), #18777, .T. ) ;
#2165=CARTESIAN_POINT ( 'NONE',  ( -3.458734124999999437, 0.000000000000000000, 16.68750000136560629 ) ) ;
#2174=CARTESIAN_POINT ( 'NONE',  ( 1.872352939448454495E-15, -3.458734125000000770, 12.93750000136560629 ) ) ;
#2180=CARTESIAN_POINT ( 'NONE',  ( -3.458734124999998105, 1.432654583217640276, 10.37500000136560629 ) ) ;
#2181=CARTESIAN_POINT ( 'NONE',  ( 2.828427124746191179, 2.828427124746190291, 15.75000000273119660 ) ) ;
#2193=DIRECTION ( 'NONE',  ( -0.000000000000000000, -0.000000000000000000, -1.000000000000000000 ) ) ;
#2195=CARTESIAN_POINT ( 'NONE',  ( 1.656854249492381470, 4.000000000000000000, 13.68750000000001066 ) ) ;
#2210=CARTESIAN_POINT ( 'NONE',  ( 1.872352939448454495E-15, -3.458734125000000770, 16.93750000136560629 ) ) ;
#2213=LINE ( 'NONE', #10993, #18583 ) ;
#2214=ORIENTED_EDGE ( 'NONE', *, *, #14206, .F. ) ;
#2225=EDGE_LOOP ( 'NONE', ( #9888, #800, #7702, #7024 ) ) ;
#2227=EDGE_LOOP ( 'NONE', ( #12808, #7264, #9979, #16944 ) ) ;
#2237=CARTESIAN_POINT ( 'NONE',  ( -2.828427124746188515, -2.828427124746190735, 13.25000000273119660 ) ) ;
#2248=DIRECTION ( 'NONE',  ( -0.000000000000000000, 1.000000000000000000, -0.000000000000000000 ) ) ;
#2250=ORIENTED_EDGE ( 'NONE', *, *, #23464, .T. ) ;
#2255=VERTEX_POINT ( 'NONE', #10851 ) ;
#2257=VERTEX_POINT ( 'NONE', #3519 ) ;
#2258=EDGE_CURVE ( 'NONE', #2257, #1597, #4239, .T. ) ;
#2259=( BOUNDED_CURVE ( )  B_SPLINE_CURVE ( 2, ( #11515, #18535, #2122, #4168, #18787, #4524, #11860, #17237, #22962 ),
 .UNSPECIFIED., .F., .F. ) 
 B_SPLINE_CURVE_WITH_KNOTS ( ( 3, 2, 2, 2, 3 ),
 ( 0.7500000000000000000, 0.7624999999999999556, 0.7750000000000000222, 0.7874999999999999778, 0.8000000000000000444 ),
 .UNSPECIFIED. ) 
 CURVE ( )  GEOMETRIC_REPRESENTATION_ITEM ( )  RATIONAL_B_SPLINE_CURVE ( ( 1.000000000000000000, 0.9238795325112867385, 1.000000000000000000, 0.9238795325112867385, 1.000000000000000000, 0.9238795325112867385, 1.000000000000000000, 0.9238795325112867385, 1.000000000000000000 ) ) 
 REPRESENTATION_ITEM ( '' )  );
#2262=VECTOR ( 'NONE', #19534, 1000.000000000000000 ) ;
#2263=CARTESIAN_POINT ( 'NONE',  ( -1.656854249492379250, 4.000000000000000000, 14.81250000000001066 ) ) ;
#2269=EDGE_LOOP ( 'NONE', ( #22214, #7129, #19850, #629 ) ) ;
#2273=CARTESIAN_POINT ( 'NONE',  ( 1.025207404391860050E-15, 3.458734125000000770, 10.43750000136560629 ) ) ;
#2275=CARTESIAN_POINT ( 'NONE',  ( 1.432654583217641164, 3.458734125000000326, 12.12500000136560629 ) ) ;
#2281=CARTESIAN_POINT ( 'NONE',  ( 4.000000000000000888, 1.656854249492381248, 12.56250000000001243 ) ) ;
#2282=CARTESIAN_POINT ( 'NONE',  ( 1.432654583217643163, -3.458734124999999437, 12.75000000136560629 ) ) ;
#2296=CARTESIAN_POINT ( 'NONE',  ( 3.458734125000002546, -1.432654583217639610, 15.12500000136560807 ) ) ;
#2298=VECTOR ( 'NONE', #6085, 1000.000000000000000 ) ;
#2309=ADVANCED_FACE ( 'NONE', ( #1825 ), #5623, .T. ) ;
#2310=CARTESIAN_POINT ( 'NONE',  ( -2.445694354108818303, -2.445694354108820523, 10.56250000136560452 ) ) ;
#2311=CARTESIAN_POINT ( 'NONE',  ( -2.828427124746189403, 2.828427124746190291, 15.00000000273119660 ) ) ;
#2322=CARTESIAN_POINT ( 'NONE',  ( 2.828427124746191179, 2.828427124746190291, 12.62500000000001066 ) ) ;
#2332=CARTESIAN_POINT ( 'NONE',  ( 19.99999999999999289, -9.999999999999964473, -20.00000000000000355 ) ) ;
#2336=CARTESIAN_POINT ( 'NONE',  ( 2.445694354108822299, -2.445694354108820079, 15.06250000136560452 ) ) ;
#2357=CARTESIAN_POINT ( 'NONE',  ( 1.656854249492384135, -3.999999999999999112, 12.43750000273119838 ) ) ;
#2359=( BOUNDED_CURVE ( )  B_SPLINE_CURVE ( 2, ( #14711, #16604, #9205, #14827, #183, #9429, #427, #11480, #5818 ),
 .UNSPECIFIED., .F., .F. ) 
 B_SPLINE_CURVE_WITH_KNOTS ( ( 3, 2, 2, 2, 3 ),
 ( 0.2999999999999999889, 0.3125000000000000000, 0.3250000000000000111, 0.3375000000000000222, 0.3499999999999999778 ),
 .UNSPECIFIED. ) 
 CURVE ( )  GEOMETRIC_REPRESENTATION_ITEM ( )  RATIONAL_B_SPLINE_CURVE ( ( 1.000000000000000000, 0.9238795325112867385, 1.000000000000000000, 0.9238795325112867385, 1.000000000000000000, 0.9238795325112867385, 1.000000000000000000, 0.9238795325112867385, 1.000000000000000000 ) ) 
 REPRESENTATION_ITEM ( '' )  );
#2362=CARTESIAN_POINT ( 'NONE',  ( 3.458734125000001214, 1.432654583217640498, 17.00000000136560629 ) ) ;
#2363=CARTESIAN_POINT ( 'NONE',  ( 4.000000000000000888, 4.898587196589412829E-16, 10.62500000273119660 ) ) ;
#2365=FACE_OUTER_BOUND ( 'NONE', #7378, .T. ) ;
#2377=FACE_OUTER_BOUND ( 'NONE', #1830, .T. ) ;
#2381=CARTESIAN_POINT ( 'NONE',  ( 4.000000000000000888, 1.656854249492381248, 18.68750000273119483 ) ) ;
#2382=CARTESIAN_POINT ( 'NONE',  ( -3.999999999999999112, 1.656854249492380804, 12.93750000000001243 ) ) ;
#2384=LINE ( 'NONE', #4421, #6863 ) ;
#2391=CARTESIAN_POINT ( 'NONE',  ( 3.458734125000002102, -1.432654583217639610, 13.87500000136560452 ) ) ;
#2397=CARTESIAN_POINT ( 'NONE',  ( 2.445694354108821855, -2.445694354108820079, 10.81250000136560452 ) ) ;
#2401=DIRECTION ( 'NONE',  ( -0.000000000000000000, 1.000000000000000000, -0.000000000000000000 ) ) ;
#2410=CARTESIAN_POINT ( 'NONE',  ( -1.432654583217639832, -3.458734125000000326, 16.87500000136560629 ) ) ;
#2414=VECTOR ( 'NONE', #8432, 1000.000000000000000 ) ;
#2422=CARTESIAN_POINT ( 'NONE',  ( -2.828427124746189403, 2.828427124746190291, 17.00000000273119838 ) ) ;
#2432=CARTESIAN_POINT ( 'NONE',  ( 2.828427124746192067, -2.828427124746189847, 13.37500000000001243 ) ) ;
#2439=DIRECTION ( 'NONE',  ( -1.000000000000000000, 0.000000000000000000, 0.000000000000000000 ) ) ;
#2442=CARTESIAN_POINT ( 'NONE',  ( -3.999999999999998224, -1.656854249492383024, 11.06250000000001066 ) ) ;
#2447=CARTESIAN_POINT ( 'NONE',  ( 3.458734125000001658, 4.235727675282972223E-16, 14.18750000136560629 ) ) ;
#2474=CARTESIAN_POINT ( 'NONE',  ( 1.432654583217643163, -3.458734124999999437, 17.75000000136560274 ) ) ;
#2484=CARTESIAN_POINT ( 'NONE',  ( -1.656854249492379472, 4.000000000000000000, 14.93750000273119660 ) ) ;
#2487=CARTESIAN_POINT ( 'NONE',  ( -1.393473772768861529, 3.889074120053769512, 9.929297958371448019 ) ) ;
#2489=LINE ( 'NONE', #19017, #21338 ) ;
#2491=CARTESIAN_POINT ( 'NONE',  ( 4.000000000000000888, 1.656854249492381248, 17.56250000000001066 ) ) ;
#2493=CARTESIAN_POINT ( 'NONE',  ( 2.828427124746191179, 2.828427124746190291, 12.62500000000001066 ) ) ;
#2506=CARTESIAN_POINT ( 'NONE',  ( 3.458734125000002102, -1.432654583217639610, 14.87500000136560807 ) ) ;
#2512=CARTESIAN_POINT ( 'NONE',  ( -3.458734124999998993, 1.432654583217640276, 10.37500000136560629 ) ) ;
#2516=CARTESIAN_POINT ( 'NONE',  ( 1.656854249492381470, 4.000000000000000000, 15.81250000273119660 ) ) ;
#2517=ORIENTED_EDGE ( 'NONE', *, *, #19916, .F. ) ;
#2524=CARTESIAN_POINT ( 'NONE',  ( -1.432654583217639832, -3.458734125000000326, 17.87500000136560274 ) ) ;
#2534=CARTESIAN_POINT ( 'NONE',  ( 3.458734125000002102, -1.432654583217639610, 11.87500000136560629 ) ) ;
#2535=CARTESIAN_POINT ( 'NONE',  ( 9.920644283265380691E-16, 4.000000000000000000, 11.87500000273119660 ) ) ;
#2538=CARTESIAN_POINT ( 'NONE',  ( -3.999999999999999112, 1.656854249492380582, 17.06250000273120193 ) ) ;
#2544=CARTESIAN_POINT ( 'NONE',  ( 4.000000000000001776, -1.656854249492379694, 14.43750000000001066 ) ) ;
#2551=FACE_OUTER_BOUND ( 'NONE', #2227, .T. ) ;
#2559=CARTESIAN_POINT ( 'NONE',  ( -2.445694354108819191, 2.445694354108820523, 10.56250000136560629 ) ) ;
#2591=VECTOR ( 'NONE', #22429, 1000.000000000000000 ) ;
#2592=EDGE_CURVE ( 'NONE', #158, #13665, #7029, .T. ) ;
#2597=EDGE_CURVE ( 'NONE', #5522, #17674, #3025, .T. ) ;
#2616=CARTESIAN_POINT ( 'NONE',  ( -1.656854249492379472, 4.000000000000000000, 11.81250000000001066 ) ) ;
#2622=VECTOR ( 'NONE', #15472, 1000.000000000000000 ) ;
#2624=CARTESIAN_POINT ( 'NONE',  ( -1.432654583217639610, -3.458734124999999882, 12.62500000136560629 ) ) ;
#2631=CARTESIAN_POINT ( 'NONE',  ( 9.920644283265380691E-16, 4.000000000000000000, 15.75000000000001066 ) ) ;
#2646=( BOUNDED_CURVE ( )  B_SPLINE_CURVE ( 2, ( #1975, #18162, #5702, #16722, #16851, #185, #23670, #7286, #21859 ),
 .UNSPECIFIED., .F., .F. ) 
 B_SPLINE_CURVE_WITH_KNOTS ( ( 3, 2, 2, 2, 3 ),
 ( 0.6999999999999999556, 0.7125000000000000222, 0.7249999999999999778, 0.7375000000000000444, 0.7500000000000000000 ),
 .UNSPECIFIED. ) 
 CURVE ( )  GEOMETRIC_REPRESENTATION_ITEM ( )  RATIONAL_B_SPLINE_CURVE ( ( 1.000000000000000000, 0.9238795325112867385, 1.000000000000000000, 0.9238795325112867385, 1.000000000000000000, 0.9238795325112867385, 1.000000000000000000, 0.9238795325112867385, 1.000000000000000000 ) ) 
 REPRESENTATION_ITEM ( '' )  );
#2648=CARTESIAN_POINT ( 'NONE',  ( -1.432654583217639832, -3.458734125000000326, 14.87500000136560807 ) ) ;
#2661=CARTESIAN_POINT ( 'NONE',  ( -1.656854249492380138, -3.999999999999999112, 11.31250000273119660 ) ) ;
#2676=EDGE_CURVE ( 'NONE', #8667, #10092, #18661, .T. ) ;
#2679=EDGE_LOOP ( 'NONE', ( #21500, #20742, #17797, #5032 ) ) ;
#2685=CARTESIAN_POINT ( 'NONE',  ( 4.000000000000001776, -1.656854249492379694, 15.43750000000001066 ) ) ;
#2686=CARTESIAN_POINT ( 'NONE',  ( -1.432654583217639832, -3.458734125000000326, 17.87500000136560274 ) ) ;
#2693=CARTESIAN_POINT ( 'NONE',  ( 1.025207404391860050E-15, 3.458734125000000770, 12.43750000136560629 ) ) ;
#2697=PLANE ( 'NONE',  #8229 ) ;
#2705=VERTEX_POINT ( 'NONE', #14627 ) ;
#2707=VECTOR ( 'NONE', #7921, 1000.000000000000000 ) ;
#2715=CARTESIAN_POINT ( 'NONE',  ( -2.445694354108818303, -2.445694354108820523, 17.56250000136560274 ) ) ;
#2744=CARTESIAN_POINT ( 'NONE',  ( -3.458734124999998993, -1.432654583217642497, 14.50000000136560629 ) ) ;
#2750=CARTESIAN_POINT ( 'NONE',  ( -3.458734124999998993, -1.432654583217642497, 10.50000000136560452 ) ) ;
#2754=ORIENTED_EDGE ( 'NONE', *, *, #11123, .T. ) ;
#2760=CARTESIAN_POINT ( 'NONE',  ( 3.458734125000001658, 1.432654583217640498, 14.25000000136560629 ) ) ;
#2775=CARTESIAN_POINT ( 'NONE',  ( 2.828427124746191179, 2.828427124746190291, 13.75000000273119483 ) ) ;
#2776=CARTESIAN_POINT ( 'NONE',  ( -2.762848947613220307, 4.746226468750993632, -26.84672628368516811 ) ) ;
#2795=CARTESIAN_POINT ( 'NONE',  ( 2.828427124746192067, -2.828427124746189847, 15.37500000000001066 ) ) ;
#2798=CARTESIAN_POINT ( 'NONE',  ( 1.971781867644420635E-15, -4.000000000000000000, 13.37500000273119660 ) ) ;
#2806=CARTESIAN_POINT ( 'NONE',  ( 1.432654583217641386, 3.458734125000000770, 11.37500000136560452 ) ) ;
#2811=ORIENTED_EDGE ( 'NONE', *, *, #3331, .F. ) ;
#2817=AXIS2_PLACEMENT_3D ( 'NONE', #1503, #21609, #1146 ) ;
#2819=ORIENTED_EDGE ( 'NONE', *, *, #20584, .F. ) ;
#2820=PRESENTATION_STYLE_ASSIGNMENT (( #19692 ) ) ;
#2844=VECTOR ( 'NONE', #17384, 1000.000000000000000 ) ;
#2846=LINE ( 'NONE', #21044, #19902 ) ;
#2854=CARTESIAN_POINT ( 'NONE',  ( 3.458734125000001658, 4.235727675282972223E-16, 17.18750000136560629 ) ) ;
#2860=CARTESIAN_POINT ( 'NONE',  ( 4.000000000000000888, 4.898587196589412829E-16, 18.62500000273119483 ) ) ;
#2873=CARTESIAN_POINT ( 'NONE',  ( 2.445694354108822299, -2.445694354108820079, 14.06250000136560629 ) ) ;
#2888=CARTESIAN_POINT ( 'NONE',  ( -3.999999999999999112, 1.656854249492380804, 11.06250000273119660 ) ) ;
#2892=ORIENTED_EDGE ( 'NONE', *, *, #8366, .T. ) ;
#2908=CARTESIAN_POINT ( 'NONE',  ( 3.458734125000001658, 1.432654583217640498, 18.25000000136560629 ) ) ;
#2909=CARTESIAN_POINT ( 'NONE',  ( 9.920644283265380691E-16, 4.000000000000000000, 13.87500000273119483 ) ) ;
#2916=CARTESIAN_POINT ( 'NONE',  ( -1.432654583217639166, 3.458734125000000770, 10.50000000136560629 ) ) ;
#2942=CARTESIAN_POINT ( 'NONE',  ( -1.432654583217638944, 3.458734125000000326, 13.25000000136560274 ) ) ;
#2946=ORIENTED_EDGE ( 'NONE', *, *, #13820, .F. ) ;
#2953=CARTESIAN_POINT ( 'NONE',  ( -3.999999999999999112, 0.000000000000000000, 14.12500000273119660 ) ) ;
#2961=DIRECTION ( 'NONE',  ( 0.000000000000000000, -0.000000000000000000, -1.000000000000000000 ) ) ;
#2965=CARTESIAN_POINT ( 'NONE',  ( 4.000000000000000888, 1.656854249492381248, 11.56250000000001066 ) ) ;
#2968=B_SPLINE_CURVE_WITH_KNOTS ( 'NONE', 1,
 ( #8693, #17902 ),
 .UNSPECIFIED., .F., .F.,
 ( 2, 2 ),
 ( 0.000000000000000000, 1.000000000000000000 ),
 .UNSPECIFIED. ) ;
#2973=CARTESIAN_POINT ( 'NONE',  ( 1.432654583217641164, 3.458734125000000326, 11.12500000136560452 ) ) ;
#2983=CARTESIAN_POINT ( 'NONE',  ( -0.8800590352214046064, 5.420839058164813373, 10.00000000000000888 ) ) ;
#2988=ORIENTED_EDGE ( 'NONE', *, *, #5991, .T. ) ;
#2992=VERTEX_POINT ( 'NONE', #3313 ) ;
#2993=CARTESIAN_POINT ( 'NONE',  ( -3.458734124999999437, 1.432654583217640498, 14.62500000136560629 ) ) ;
#2997=CYLINDRICAL_SURFACE ( 'NONE', #18292, 4.000000000000000000 ) ;
#3004=CIRCLE ( 'NONE', #19068, 4.999999999999999112 ) ;
#3008=CARTESIAN_POINT ( 'NONE',  ( 3.458734125000001214, 4.235727675282971730E-16, 15.93750000136560629 ) ) ;
#3022=DIRECTION ( 'NONE',  ( -1.000000000000000000, 0.000000000000000000, 1.982541115402065110E-16 ) ) ;
#3025=( BOUNDED_CURVE ( )  B_SPLINE_CURVE ( 2, ( #8882, #8751, #14270, #21532, #3343, #1541, #10685, #17961, #16175 ),
 .UNSPECIFIED., .F., .F. ) 
 B_SPLINE_CURVE_WITH_KNOTS ( ( 3, 2, 2, 2, 3 ),
 ( 0.8000000000000000444, 0.8125000000000000000, 0.8249999999999999556, 0.8375000000000000222, 0.8499999999999999778 ),
 .UNSPECIFIED. ) 
 CURVE ( )  GEOMETRIC_REPRESENTATION_ITEM ( )  RATIONAL_B_SPLINE_CURVE ( ( 1.000000000000000000, 0.9238795325112867385, 1.000000000000000000, 0.9238795325112867385, 1.000000000000000000, 0.9238795325112867385, 1.000000000000000000, 0.9238795325112867385, 1.000000000000000000 ) ) 
 REPRESENTATION_ITEM ( '' )  );
#3033=CARTESIAN_POINT ( 'NONE',  ( 2.445694354108822299, -2.445694354108820079, 15.06250000136560452 ) ) ;
#3035=CARTESIAN_POINT ( 'NONE',  ( 1.656854249492384135, -3.999999999999999112, 15.43750000273119660 ) ) ;
#3042=CARTESIAN_POINT ( 'NONE',  ( 1.432654583217643163, -3.458734124999999882, 12.00000000136560452 ) ) ;
#3046=EDGE_LOOP ( 'NONE', ( #15090, #17739, #20445, #10941, #8859, #7784 ) ) ;
#3057=CARTESIAN_POINT ( 'NONE',  ( 0.000000000000000000, 0.000000000000000000, 20.00000000000001066 ) ) ;
#3061=AXIS2_PLACEMENT_3D ( 'NONE', #19098, #8899, #20874 ) ;
#3063=CARTESIAN_POINT ( 'NONE',  ( -1.656854249492379250, 4.000000000000000000, 11.81250000000001066 ) ) ;
#3071=CARTESIAN_POINT ( 'NONE',  ( -15.00000000000001066, -10.00000000000000000, -49.99999999999999289 ) ) ;
#3075=CARTESIAN_POINT ( 'NONE',  ( 3.458734125000001214, 1.432654583217640498, 16.00000000136560629 ) ) ;
#3089=DIRECTION ( 'NONE',  ( -1.000000000000000000, 0.000000000000000000, 0.000000000000000000 ) ) ;
#3098=DIRECTION ( 'NONE',  ( 1.000000000000000000, 0.000000000000000000, 0.000000000000000000 ) ) ;
#3103=CARTESIAN_POINT ( 'NONE',  ( 3.458734125000001658, 1.432654583217640498, 18.25000000136560629 ) ) ;
#3105=EDGE_CURVE ( 'NONE', #1597, #15665, #23422, .T. ) ;
#3110=DIRECTION ( 'NONE',  ( 0.000000000000000000, 0.000000000000000000, -1.000000000000000000 ) ) ;
#3111=CARTESIAN_POINT ( 'NONE',  ( 0.000000000000000000, 0.000000000000000000, 0.000000000000000000 ) ) ;
#3121=CARTESIAN_POINT ( 'NONE',  ( 2.445694354108822299, -2.445694354108820079, 11.06250000136560452 ) ) ;
#3133=CARTESIAN_POINT ( 'NONE',  ( 3.458734125000001214, 4.235727675282971730E-16, 18.93750000136560629 ) ) ;
#3140=VERTEX_POINT ( 'NONE', #5822 ) ;
#3145=EDGE_LOOP ( 'NONE', ( #7836, #14584, #6555, #11805 ) ) ;
#3150=CARTESIAN_POINT ( 'NONE',  ( 1.025207404391860050E-15, 3.458734125000000770, 14.43750000136560452 ) ) ;
#3165=DIRECTION ( 'NONE',  ( -1.000000000000000000, 0.000000000000000000, 0.000000000000000000 ) ) ;
#3185=CARTESIAN_POINT ( 'NONE',  ( 2.445694354108821411, 2.445694354108820523, 14.06250000136560452 ) ) ;
#3203=EDGE_CURVE ( 'NONE', #13418, #17227, #7176, .T. ) ;
#3212=LINE ( 'NONE', #3333, #21746 ) ;
#3214=CARTESIAN_POINT ( 'NONE',  ( 3.458734125000002546, -1.432654583217639610, 18.12500000136560274 ) ) ;
#3228=EDGE_CURVE ( 'NONE', #7815, #1384, #5586, .T. ) ;
#3234=CARTESIAN_POINT ( 'NONE',  ( -1.432654583217639832, -3.458734125000000326, 10.87500000136560452 ) ) ;
#3250=CARTESIAN_POINT ( 'NONE',  ( 1.432654583217643163, -3.458734124999999437, 18.75000000136560274 ) ) ;
#3253=DIRECTION ( 'NONE',  ( 0.000000000000000000, 1.000000000000000000, 0.000000000000000000 ) ) ;
#3273=( BOUNDED_SURFACE ( )  B_SPLINE_SURFACE ( 1, 2, ( 
 ( #1934, #23624, #5653, #7236, #139, #5421, #9276, #16561, #7468, #14788, #22036, #12987, #11308, #13222, #7713, #11433, #11670, #20726, #20608, #15141, #614, #9860, #18939, #8069, #22163, #17158, #5780, #15028, #15260, #2524, #18705, #6014, #20364, #7940, #4330, #19057, #13341, #18584, #11784, #251, #4449, #13571, #20840, #3974, #22282, #2410, #736, #15384, #2165, #22406, #9743, #6252, #7823, #22528, #22647, #4217, #5898, #9386, #16680, #14905, #6140, #11556, #7587, #13108, #18825, #13465, #17037, #9503, #16800, #381, #20490, #4091, #9633, #2296, #16923, #500, #19177, #2648, #20952, #5041, #17280, #2993, #23228, #12372, #14162, #4573, #8535, #2760, #6838, #6375, #2873, #19284, #23006, #4684, #848, #8421, #10221, #9989, #11907, #1197, #6495, #15945, #21425, #10461, #961, #12017, #8179, #21182, #22763, #13928, #15841, #10103, #13817, #8294, #17511, #4920, #14035, #4799, #15734, #15614, #15493, #12255, #21297, #13690, #1309, #17392, #22884, #21076, #19523, #1080, #6612, #12132, #17743, #19398, #10346, #17635, #23111, #6723, #3121, #8645, #10926, #3234, #19985, #14755, #5394, #14524, #3699, #9129, #16419 ),
 ( #21543, #5626, #7441, #14282, #5152, #16185, #10695, #19875, #16308, #12494, #1906, #19755, #1671, #20099, #1423, #11039, #5273, #7083, #12734, #14400, #1552, #18207, #18324, #18088, #108, #22011, #17974, #3588, #6965, #21787, #1785, #8766, #17854, #1, #19636, #3355, #10583, #9249, #16533, #16070, #12615, #7332, #21663, #14638, #23360, #8891, #23474, #3479, #10816, #23595, #21898, #9012, #7208, #5507, #12840, #698, #11164, #11275, #16647, #18438, #3828, #20576, #14875, #9604, #11528, #13192, #2136, #9712, #18549, #9356, #18674, #4062, #225, #7796, #22619, #22490, #5750, #15002, #18907, #8033, #9829, #7554, #11640, #2263, #16896, #7684, #13435, #22253, #2015, #3941, #12957, #5864, #22133, #16768, #15111, #18799, #13079, #20219, #471, #20456, #20335, #22371, #20697, #6103, #582, #4304, #17123, #15352, #11396, #5982, #9471, #13306, #4184, #2382, #350, #17008, #7908, #15225, #2493, #821, #16244, #15895, #12315, #11876, #10761, #8837, #17916, #9955, #5213, #18036, #1613, #3063, #16135, #19466, #17249, #17799, #14341, #14101, #16011, #23297, #6224, #8153, #1496, #8955, #21482, #13543, #6907, #20812, #14227 ) ),
 .UNSPECIFIED., .F., .F., .F. ) 
 B_SPLINE_SURFACE_WITH_KNOTS ( ( 2, 2 ),
 ( 3, 2, 2, 2, 2, 2, 2, 2, 2, 2, 2, 2, 2, 2, 2, 2, 2, 2, 2, 2, 2, 2, 2, 2, 2, 2, 2, 2, 2, 2, 2, 2, 2, 2, 2, 2, 2, 2, 2, 2, 2, 2, 2, 2, 2, 2, 2, 2, 2, 2, 2, 2, 2, 2, 2, 2, 2, 2, 2, 2, 2, 2, 2, 2, 2, 2, 2, 2, 2, 2, 2, 2, 2, 2, 3 ),
 ( 0.000000000000000000, 1.000000000000000000 ),
 ( 0.000000000000000000, 0.01250000000000000069, 0.02500000000000000139, 0.03749999999999999861, 0.05000000000000000278, 0.06250000000000000000, 0.07499999999999999722, 0.08749999999999999445, 0.1000000000000000056, 0.1125000000000000028, 0.1250000000000000000, 0.1375000000000000111, 0.1499999999999999944, 0.1625000000000000056, 0.1749999999999999889, 0.1875000000000000000, 0.2000000000000000111, 0.2124999999999999944, 0.2250000000000000056, 0.2374999999999999889, 0.2500000000000000000, 0.2625000000000000111, 0.2750000000000000222, 0.2874999999999999778, 0.2999999999999999889, 0.3125000000000000000, 0.3250000000000000111, 0.3375000000000000222, 0.3499999999999999778, 0.3624999999999999889, 0.3750000000000000000, 0.3875000000000000111, 0.4000000000000000222, 0.4124999999999999778, 0.4249999999999999889, 0.4375000000000000000, 0.4500000000000000111, 0.4625000000000000222, 0.4749999999999999778, 0.4874999999999999889, 0.5000000000000000000, 0.5124999999999999556, 0.5250000000000000222, 0.5374999999999999778, 0.5500000000000000444, 0.5625000000000000000, 0.5749999999999999556, 0.5875000000000000222, 0.5999999999999999778, 0.6125000000000000444, 0.6250000000000000000, 0.6374999999999999556, 0.6500000000000000222, 0.6624999999999999778, 0.6750000000000000444, 0.6875000000000000000, 0.6999999999999999556, 0.7125000000000000222, 0.7249999999999999778, 0.7375000000000000444, 0.7500000000000000000, 0.7624999999999999556, 0.7750000000000000222, 0.7874999999999999778, 0.8000000000000000444, 0.8125000000000000000, 0.8249999999999999556, 0.8375000000000000222, 0.8499999999999999778, 0.8625000000000000444, 0.8750000000000000000, 0.8874999999999999556, 0.9000000000000000222, 0.9124999999999999778, 0.9250000000000000444 ),
 .UNSPECIFIED. ) 
 GEOMETRIC_REPRESENTATION_ITEM ( )  RATIONAL_B_SPLINE_SURFACE ( (
 ( 1.000000000000000000, 0.9238795325112867385, 1.000000000000000000, 0.9238795325112867385, 1.000000000000000000, 0.9238795325112867385, 1.000000000000000000, 0.9238795325112867385, 1.000000000000000000, 0.9238795325112867385, 1.000000000000000000, 0.9238795325112867385, 1.000000000000000000, 0.9238795325112867385, 1.000000000000000000, 0.9238795325112867385, 1.000000000000000000, 0.9238795325112867385, 1.000000000000000000, 0.9238795325112867385, 1.000000000000000000, 0.9238795325112867385, 1.000000000000000000, 0.9238795325112867385, 1.000000000000000000, 0.9238795325112867385, 1.000000000000000000, 0.9238795325112867385, 1.000000000000000000, 0.9238795325112867385, 1.000000000000000000, 0.9238795325112867385, 1.000000000000000000, 0.9238795325112867385, 1.000000000000000000, 0.9238795325112867385, 1.000000000000000000, 0.9238795325112867385, 1.000000000000000000, 0.9238795325112867385, 1.000000000000000000, 0.9238795325112867385, 1.000000000000000000, 0.9238795325112867385, 1.000000000000000000, 0.9238795325112867385, 1.000000000000000000, 0.9238795325112867385, 1.000000000000000000, 0.9238795325112867385, 1.000000000000000000, 0.9238795325112867385, 1.000000000000000000, 0.9238795325112867385, 1.000000000000000000, 0.9238795325112867385, 1.000000000000000000, 0.9238795325112867385, 1.000000000000000000, 0.9238795325112867385, 1.000000000000000000, 0.9238795325112867385, 1.000000000000000000, 0.9238795325112867385, 1.000000000000000000, 0.9238795325112867385, 1.000000000000000000, 0.9238795325112867385, 1.000000000000000000, 0.9238795325112867385, 1.000000000000000000, 0.9238795325112867385, 1.000000000000000000, 0.9238795325112867385, 1.000000000000000000, 0.9238795325112867385, 1.000000000000000000, 0.9238795325112867385, 1.000000000000000000, 0.9238795325112867385, 1.000000000000000000, 0.9238795325112867385, 1.000000000000000000, 0.9238795325112867385, 1.000000000000000000, 0.9238795325112867385, 1.000000000000000000, 0.9238795325112867385, 1.000000000000000000, 0.9238795325112867385, 1.000000000000000000, 0.9238795325112867385, 1.000000000000000000, 0.9238795325112867385, 1.000000000000000000, 0.9238795325112867385, 1.000000000000000000, 0.9238795325112867385, 1.000000000000000000, 0.9238795325112867385, 1.000000000000000000, 0.9238795325112867385, 1.000000000000000000, 0.9238795325112867385, 1.000000000000000000, 0.9238795325112867385, 1.000000000000000000, 0.9238795325112867385, 1.000000000000000000, 0.9238795325112867385, 1.000000000000000000, 0.9238795325112867385, 1.000000000000000000, 0.9238795325112867385, 1.000000000000000000, 0.9238795325112867385, 1.000000000000000000, 0.9238795325112867385, 1.000000000000000000, 0.9238795325112867385, 1.000000000000000000, 0.9238795325112867385, 1.000000000000000000, 0.9238795325112867385, 1.000000000000000000, 0.9238795325112867385, 1.000000000000000000, 0.9238795325112867385, 1.000000000000000000, 0.9238795325112867385, 1.000000000000000000, 0.9238795325112867385, 1.000000000000000000, 0.9238795325112867385, 1.000000000000000000, 0.9238795325112867385, 1.000000000000000000, 0.9238795325112867385, 1.000000000000000000, 0.9238795325112867385, 1.000000000000000000, 0.9238795325112867385, 1.000000000000000000, 0.9238795325112867385, 1.000000000000000000, 0.9238795325112867385, 1.000000000000000000, 0.9238795325112867385, 1.000000000000000000),
 ( 1.000000000000000000, 0.9238795325112867385, 1.000000000000000000, 0.9238795325112867385, 1.000000000000000000, 0.9238795325112867385, 1.000000000000000000, 0.9238795325112867385, 1.000000000000000000, 0.9238795325112867385, 1.000000000000000000, 0.9238795325112867385, 1.000000000000000000, 0.9238795325112867385, 1.000000000000000000, 0.9238795325112867385, 1.000000000000000000, 0.9238795325112867385, 1.000000000000000000, 0.9238795325112867385, 1.000000000000000000, 0.9238795325112867385, 1.000000000000000000, 0.9238795325112867385, 1.000000000000000000, 0.9238795325112867385, 1.000000000000000000, 0.9238795325112867385, 1.000000000000000000, 0.9238795325112867385, 1.000000000000000000, 0.9238795325112867385, 1.000000000000000000, 0.9238795325112867385, 1.000000000000000000, 0.9238795325112867385, 1.000000000000000000, 0.9238795325112867385, 1.000000000000000000, 0.9238795325112867385, 1.000000000000000000, 0.9238795325112867385, 1.000000000000000000, 0.9238795325112867385, 1.000000000000000000, 0.9238795325112867385, 1.000000000000000000, 0.9238795325112867385, 1.000000000000000000, 0.9238795325112867385, 1.000000000000000000, 0.9238795325112867385, 1.000000000000000000, 0.9238795325112867385, 1.000000000000000000, 0.9238795325112867385, 1.000000000000000000, 0.9238795325112867385, 1.000000000000000000, 0.9238795325112867385, 1.000000000000000000, 0.9238795325112867385, 1.000000000000000000, 0.9238795325112867385, 1.000000000000000000, 0.9238795325112867385, 1.000000000000000000, 0.9238795325112867385, 1.000000000000000000, 0.9238795325112867385, 1.000000000000000000, 0.9238795325112867385, 1.000000000000000000, 0.9238795325112867385, 1.000000000000000000, 0.9238795325112867385, 1.000000000000000000, 0.9238795325112867385, 1.000000000000000000, 0.9238795325112867385, 1.000000000000000000, 0.9238795325112867385, 1.000000000000000000, 0.9238795325112867385, 1.000000000000000000, 0.9238795325112867385, 1.000000000000000000, 0.9238795325112867385, 1.000000000000000000, 0.9238795325112867385, 1.000000000000000000, 0.9238795325112867385, 1.000000000000000000, 0.9238795325112867385, 1.000000000000000000, 0.9238795325112867385, 1.000000000000000000, 0.9238795325112867385, 1.000000000000000000, 0.9238795325112867385, 1.000000000000000000, 0.9238795325112867385, 1.000000000000000000, 0.9238795325112867385, 1.000000000000000000, 0.9238795325112867385, 1.000000000000000000, 0.9238795325112867385, 1.000000000000000000, 0.9238795325112867385, 1.000000000000000000, 0.9238795325112867385, 1.000000000000000000, 0.9238795325112867385, 1.000000000000000000, 0.9238795325112867385, 1.000000000000000000, 0.9238795325112867385, 1.000000000000000000, 0.9238795325112867385, 1.000000000000000000, 0.9238795325112867385, 1.000000000000000000, 0.9238795325112867385, 1.000000000000000000, 0.9238795325112867385, 1.000000000000000000, 0.9238795325112867385, 1.000000000000000000, 0.9238795325112867385, 1.000000000000000000, 0.9238795325112867385, 1.000000000000000000, 0.9238795325112867385, 1.000000000000000000, 0.9238795325112867385, 1.000000000000000000, 0.9238795325112867385, 1.000000000000000000, 0.9238795325112867385, 1.000000000000000000, 0.9238795325112867385, 1.000000000000000000, 0.9238795325112867385, 1.000000000000000000, 0.9238795325112867385, 1.000000000000000000, 0.9238795325112867385, 1.000000000000000000) ) ) 
 REPRESENTATION_ITEM ( '' )  SURFACE ( )  );
#3274=CARTESIAN_POINT ( 'NONE',  ( 1.432654583217643163, -3.458734124999999882, 16.00000000136560629 ) ) ;
#3286=VERTEX_POINT ( 'NONE', #13150 ) ;
#3301=ORIENTED_EDGE ( 'NONE', *, *, #15537, .T. ) ;
#3302=EDGE_CURVE ( 'NONE', #17674, #15665, #21861, .T. ) ;
#3303=CARTESIAN_POINT ( 'NONE',  ( 19.99999999999998934, 9.999999999999964473, -50.00000000000000000 ) ) ;
#3307=CARTESIAN_POINT ( 'NONE',  ( -3.458734124999998993, 0.000000000000000000, 15.43750000136560452 ) ) ;
#3310=EDGE_LOOP ( 'NONE', ( #4795, #8287, #22660, #12729, #7641 ) ) ;
#3313=CARTESIAN_POINT ( 'NONE',  ( 4.000000000000000888, 4.898587196589412829E-16, 20.00000000000001066 ) ) ;
#3317=ORIENTED_EDGE ( 'NONE', *, *, #14577, .F. ) ;
#3326=DIRECTION ( 'NONE',  ( -0.000000000000000000, -0.000000000000000000, -1.000000000000000000 ) ) ;
#3331=EDGE_CURVE ( 'NONE', #2257, #7929, #16724, .T. ) ;
#3333=CARTESIAN_POINT ( 'NONE',  ( 14.99999999999995914, 15.00000000000000000, -20.00000000000000355 ) ) ;
#3336=CARTESIAN_POINT ( 'NONE',  ( -2.445694354108819191, 2.445694354108820523, 17.56250000136560274 ) ) ;
#3343=CARTESIAN_POINT ( 'NONE',  ( 9.920644283265380691E-16, 4.000000000000000000, 10.87500000273119660 ) ) ;
#3344=DIRECTION ( 'NONE',  ( 1.000000000000000000, 0.000000000000000000, 0.000000000000000000 ) ) ;
#3352=ORIENTED_EDGE ( 'NONE', *, *, #21094, .T. ) ;
#3355=CARTESIAN_POINT ( 'NONE',  ( -1.656854249492379250, 4.000000000000000000, 17.81250000000001421 ) ) ;
#3357=AXIS2_PLACEMENT_3D ( 'NONE', #6341, #15581, #17478 ) ;
#3363=EDGE_CURVE ( 'NONE', #9768, #2705, #4914, .T. ) ;
#3367=LINE ( 'NONE', #23016, #2262 ) ;
#3369=CARTESIAN_POINT ( 'NONE',  ( -2.445694354108819191, 2.445694354108820523, 19.31250000136560629 ) ) ;
#3370=DIRECTION ( 'NONE',  ( 0.000000000000000000, 0.000000000000000000, 1.000000000000000000 ) ) ;
#3376=CARTESIAN_POINT ( 'NONE',  ( 2.828427124746192067, -2.828427124746189847, 14.50000000273119660 ) ) ;
#3377=ORIENTED_EDGE ( 'NONE', *, *, #3793, .T. ) ;
#3385=ORIENTED_EDGE ( 'NONE', *, *, #4860, .F. ) ;
#3391=CARTESIAN_POINT ( 'NONE',  ( -2.445694354108819191, 2.445694354108820523, 15.56250000136560629 ) ) ;
#3394=FACE_OUTER_BOUND ( 'NONE', #5114, .T. ) ;
#3397=CARTESIAN_POINT ( 'NONE',  ( -2.828427124746188515, -2.828427124746190735, 18.25000000273119483 ) ) ;
#3398=VECTOR ( 'NONE', #13906, 1000.000000000000000 ) ;
#3406=ORIENTED_EDGE ( 'NONE', *, *, #1894, .T. ) ;
#3412=CARTESIAN_POINT ( 'NONE',  ( 9.920644283265380691E-16, 4.000000000000000000, 17.75000000000000711 ) ) ;
#3413=ORIENTED_EDGE ( 'NONE', *, *, #23257, .T. ) ;
#3419=CARTESIAN_POINT ( 'NONE',  ( -35.00000000000000000, 7.500000000000001776, -19.99999999999998934 ) ) ;
#3426=CARTESIAN_POINT ( 'NONE',  ( -3.999999999999999112, 0.000000000000000000, 17.12500000273119838 ) ) ;
#3432=CARTESIAN_POINT ( 'NONE',  ( -1.432654583217638944, 3.458734125000000326, 16.25000000136560629 ) ) ;
#3440=ORIENTED_EDGE ( 'NONE', *, *, #16382, .F. ) ;
#3453=FACE_OUTER_BOUND ( 'NONE', #12680, .T. ) ;
#3456=CARTESIAN_POINT ( 'NONE',  ( -3.999999999999998224, -1.656854249492383246, 16.18750000273119838 ) ) ;
#3460=CARTESIAN_POINT ( 'NONE',  ( 19.99999999999998934, 9.999999999999964473, -50.00000000000000000 ) ) ;
#3477=CARTESIAN_POINT ( 'NONE',  ( 4.000000000000000888, 1.656854249492381248, 18.56250000000001421 ) ) ;
#3479=CARTESIAN_POINT ( 'NONE',  ( -3.999999999999998224, -1.656854249492383246, 17.06250000000001421 ) ) ;
#3482=CARTESIAN_POINT ( 'NONE',  ( -3.999999999999999112, 0.000000000000000000, 11.00000000000001066 ) ) ;
#3483=LINE ( 'NONE', #10819, #20187 ) ;
#3492=CARTESIAN_POINT ( 'NONE',  ( -0.6948844085414769278, 3.953085111073343594, 9.999322813920281661 ) ) ;
#3493=CARTESIAN_POINT ( 'NONE',  ( 2.445694354108821855, -2.445694354108820079, 16.81250000136560629 ) ) ;
#3497=CARTESIAN_POINT ( 'NONE',  ( 2.828427124746191179, 2.828427124746190291, 16.75000000273119838 ) ) ;
#3505=ADVANCED_FACE ( 'NONE', ( #16180 ), #23469, .F. ) ;
#3513=CARTESIAN_POINT ( 'NONE',  ( -3.458734124999999437, 1.432654583217640498, 16.62500000136560629 ) ) ;
#3516=CARTESIAN_POINT ( 'NONE',  ( -3.999999999999999112, 0.000000000000000000, -20.00000000000000000 ) ) ;
#3519=CARTESIAN_POINT ( 'NONE',  ( -2.247776618166699603, 3.308700692843501656, -19.99999999999999289 ) ) ;
#3529=CARTESIAN_POINT ( 'NONE',  ( 4.000000000000000888, 4.898587196589412829E-16, 16.50000000000001066 ) ) ;
#3544=CARTESIAN_POINT ( 'NONE',  ( -3.458734124999998993, 0.000000000000000000, 12.43750000136560629 ) ) ;
#3567=CARTESIAN_POINT ( 'NONE',  ( -3.999999999999998224, -1.656854249492383246, 18.18750000273119483 ) ) ;
#3576=CARTESIAN_POINT ( 'NONE',  ( -3.729367062499998831, 0.000000000000000000, 19.84375000068280670 ) ) ;
#3586=VERTEX_POINT ( 'NONE', #12833 ) ;
#3587=DIRECTION ( 'NONE',  ( -1.224646799147353207E-16, 0.000000000000000000, -1.000000000000000000 ) ) ;
#3588=CARTESIAN_POINT ( 'NONE',  ( 1.656854249492384135, -3.999999999999999112, 18.31250000000001421 ) ) ;
#3589=LINE ( 'NONE', #21899, #774 ) ;
#3594=CYLINDRICAL_SURFACE ( 'NONE', #4943, 4.000000000000000000 ) ;
#3595=CARTESIAN_POINT ( 'NONE',  ( -1.432654583217639610, -3.458734124999999882, 16.62500000136560629 ) ) ;
#3600=CARTESIAN_POINT ( 'NONE',  ( -2.445694354108818303, -2.445694354108820523, 15.56250000136560629 ) ) ;
#3618=CARTESIAN_POINT ( 'NONE',  ( -1.432654583217639832, -3.458734125000000326, 10.87500000136560452 ) ) ;
#3619=CARTESIAN_POINT ( 'NONE',  ( 1.971781867644420635E-15, -4.000000000000000000, 10.37500000273119660 ) ) ;
#3638=CARTESIAN_POINT ( 'NONE',  ( 4.000000000000001776, -1.656854249492379694, 16.43750000000001066 ) ) ;
#3643=LINE ( 'NONE', #5568, #9093 ) ;
#3655=CARTESIAN_POINT ( 'NONE',  ( -3.999999999999999112, 0.000000000000000000, 18.12500000273119483 ) ) ;
#3677=CARTESIAN_POINT ( 'NONE',  ( 1.656854249492381470, 4.000000000000000000, 18.81250000273119838 ) ) ;
#3685=DIRECTION ( 'NONE',  ( -1.000000000000000000, 0.000000000000000000, 0.000000000000000000 ) ) ;
#3697=CARTESIAN_POINT ( 'NONE',  ( -3.999999999999999112, 0.000000000000000000, 19.12500000273119838 ) ) ;
#3699=CARTESIAN_POINT ( 'NONE',  ( -2.445694354108819191, 2.445694354108820523, 10.56250000136560629 ) ) ;
#3703=ORIENTED_EDGE ( 'NONE', *, *, #11123, .F. ) ;
#3709=CARTESIAN_POINT ( 'NONE',  ( -2.445694354108819191, 2.445694354108820523, 18.31250000136560274 ) ) ;
#3713=CARTESIAN_POINT ( 'NONE',  ( 1.025207404391860050E-15, 3.458734125000000326, 15.18750000136560452 ) ) ;
#3734=CARTESIAN_POINT ( 'NONE',  ( 1.432654583217641386, 3.458734125000000770, 12.37500000136560629 ) ) ;
#3741=CARTESIAN_POINT ( 'NONE',  ( 4.000000000000001776, -1.656854249492379694, 14.56250000273119660 ) ) ;
#3751=CARTESIAN_POINT ( 'NONE',  ( 2.828427124746192067, -2.828427124746189847, 15.37500000000001066 ) ) ;
#3757=LINE ( 'NONE', #19815, #14156 ) ;
#3760=CIRCLE ( 'NONE', #23268, 2.649999999999989253 ) ;
#3772=CARTESIAN_POINT ( 'NONE',  ( -3.458734124999999437, 0.000000000000000000, 14.68750000136560452 ) ) ;
#3791=AXIS2_PLACEMENT_3D ( 'NONE', #1882, #19730, #16396 ) ;
#3793=EDGE_CURVE ( 'NONE', #10478, #5522, #10414, .T. ) ;
#3802=CARTESIAN_POINT ( 'NONE',  ( -1.656854249492380138, -3.999999999999999112, 18.31250000273119838 ) ) ;
#3819=ORIENTED_EDGE ( 'NONE', *, *, #14346, .T. ) ;
#3824=DIRECTION ( 'NONE',  ( -0.000000000000000000, -0.000000000000000000, -1.000000000000000000 ) ) ;
#3828=CARTESIAN_POINT ( 'NONE',  ( 1.971781867644420635E-15, -4.000000000000000000, 16.25000000000001066 ) ) ;
#3839=DIRECTION ( 'NONE',  ( -1.000000000000000000, 0.000000000000000000, 1.224646799147353207E-16 ) ) ;
#3841=CARTESIAN_POINT ( 'NONE',  ( 1.432654583217643163, -3.458734124999999437, 17.75000000136560629 ) ) ;
#3846=CARTESIAN_POINT ( 'NONE',  ( 1.872352939448454495E-15, -3.458734125000000326, 11.68750000136560629 ) ) ;
#3857=ORIENTED_EDGE ( 'NONE', *, *, #1176, .T. ) ;
#3863=CARTESIAN_POINT ( 'NONE',  ( 1.025207404391860050E-15, 3.458734125000000770, 12.43750000136560629 ) ) ;
#3869=CARTESIAN_POINT ( 'NONE',  ( 2.828427124746191179, 2.828427124746190291, 14.75000000273119660 ) ) ;
#3880=CARTESIAN_POINT ( 'NONE',  ( 2.828427124746191179, 2.828427124746190291, 15.62500000000001066 ) ) ;
#3884=LINE ( 'NONE', #16592, #12923 ) ;
#3891=CARTESIAN_POINT ( 'NONE',  ( 3.458734125000002546, -1.432654583217639610, 16.12500000136560629 ) ) ;
#3906=ORIENTED_EDGE ( 'NONE', *, *, #15603, .T. ) ;
#3913=CARTESIAN_POINT ( 'NONE',  ( -2.828427124746189403, 2.828427124746190291, 19.00000000273119838 ) ) ;
#3914=DIRECTION ( 'NONE',  ( 0.000000000000000000, 0.000000000000000000, -1.000000000000000000 ) ) ;
#3918=CARTESIAN_POINT ( 'NONE',  ( 14.99999999999996092, -15.00000000000000000, -20.00000000000000355 ) ) ;
#3921=FACE_OUTER_BOUND ( 'NONE', #7813, .T. ) ;
#3929=CARTESIAN_POINT ( 'NONE',  ( 4.000000000000000888, 4.898587196589412829E-16, 13.50000000000001066 ) ) ;
#3934=CARTESIAN_POINT ( 'NONE',  ( 4.000000000000001776, -1.656854249492379694, 16.56250000273119838 ) ) ;
#3941=CARTESIAN_POINT ( 'NONE',  ( 4.000000000000001776, -1.656854249492379694, 14.43750000000001066 ) ) ;
#3943=APPLICATION_CONTEXT ( 'automotive_design' ) ;
#3947=EDGE_LOOP ( 'NONE', ( #16861, #17027, #19713 ) ) ;
#3954=CARTESIAN_POINT ( 'NONE',  ( 1.432654583217641164, 3.458734125000000326, 17.12500000136560629 ) ) ;
#3958=ADVANCED_FACE ( 'NONE', ( #21523 ), #14383, .F. ) ;
#3960=CARTESIAN_POINT ( 'NONE',  ( 3.458734125000001214, 1.432654583217640498, 14.00000000136560629 ) ) ;
#3961=CYLINDRICAL_SURFACE ( 'NONE', #17621, 4.000000000000000000 ) ;
#3974=CARTESIAN_POINT ( 'NONE',  ( 1.432654583217643163, -3.458734124999999882, 17.00000000136560629 ) ) ;
#3979=CARTESIAN_POINT ( 'NONE',  ( -3.458734124999998105, -1.432654583217642497, 12.75000000136560629 ) ) ;
#3984=CARTESIAN_POINT ( 'NONE',  ( -1.432654583217639610, -3.458734124999999882, 11.62500000136560629 ) ) ;
#3985=CARTESIAN_POINT ( 'NONE',  ( 1.656854249492384135, -3.999999999999999112, 15.43750000273119660 ) ) ;
#3990=CARTESIAN_POINT ( 'NONE',  ( 1.236993788156008760E-15, 0.000000000000000000, 21.31370849898476649 ) ) ;
#3998=CARTESIAN_POINT ( 'NONE',  ( -1.656854249492380138, -3.999999999999999112, 12.18750000000001066 ) ) ;
#4014=CARTESIAN_POINT ( 'NONE',  ( 3.458734125000001658, 4.235727675282972223E-16, 13.18750000136560452 ) ) ;
#4017=B_SPLINE_CURVE_WITH_KNOTS ( 'NONE', 3,
 ( #1798, #3492, #5166, #18217, #10938, #14176 ),
 .UNSPECIFIED., .F., .F.,
 ( 4, 2, 4 ),
 ( 0.000000000000000000, 0.5000000000000000000, 1.000000000000000000 ),
 .UNSPECIFIED. ) ;
#4019=VERTEX_POINT ( 'NONE', #7537 ) ;
#4028=ORIENTED_EDGE ( 'NONE', *, *, #9524, .F. ) ;
#4035=CARTESIAN_POINT ( 'NONE',  ( -2.828427124746189403, 2.828427124746190291, 19.87500000000001066 ) ) ;
#4038=CARTESIAN_POINT ( 'NONE',  ( 4.000000000000000888, 4.898587196589412829E-16, 15.62500000273119660 ) ) ;
#4055=DIRECTION ( 'NONE',  ( -0.000000000000000000, -0.000000000000000000, -1.000000000000000000 ) ) ;
#4061=CARTESIAN_POINT ( 'NONE',  ( -3.999999999999999112, 1.656854249492380582, 19.06250000273120193 ) ) ;
#4062=CARTESIAN_POINT ( 'NONE',  ( 4.000000000000000888, 1.656854249492381248, 15.56250000000000888 ) ) ;
#4071=LINE ( 'NONE', #22382, #11470 ) ;
#4074=CARTESIAN_POINT ( 'NONE',  ( 3.458734125000001214, 1.432654583217640498, 17.00000000136560629 ) ) ;
#4079=CARTESIAN_POINT ( 'NONE',  ( 2.445694354108821855, -2.445694354108820079, 14.81250000136560452 ) ) ;
#4091=CARTESIAN_POINT ( 'NONE',  ( 3.458734125000001658, 1.432654583217640498, 15.25000000136560807 ) ) ;
#4107=CARTESIAN_POINT ( 'NONE',  ( -1.656854249492379250, 4.000000000000000000, 14.93750000273119660 ) ) ;
#4116=ORIENTED_EDGE ( 'NONE', *, *, #4730, .T. ) ;
#4117=CARTESIAN_POINT ( 'NONE',  ( 1.656854249492381470, 4.000000000000000000, 14.68750000000000888 ) ) ;
#4134=CARTESIAN_POINT ( 'NONE',  ( 1.432654583217641386, 3.458734125000000770, 16.37500000136560629 ) ) ;
#4137=AXIS2_PLACEMENT_3D ( 'NONE', #11913, #21187, #15846 ) ;
#4139=ORIENTED_EDGE ( 'NONE', *, *, #15537, .F. ) ;
#4154=FACE_OUTER_BOUND ( 'NONE', #20298, .T. ) ;
#4158=CARTESIAN_POINT ( 'NONE',  ( 9.920644283265380691E-16, 4.000000000000000000, 12.87500000273119660 ) ) ;
#4168=CARTESIAN_POINT ( 'NONE',  ( 1.656854249492384135, -3.999999999999999112, 12.31250000000001066 ) ) ;
#4175=CARTESIAN_POINT ( 'NONE',  ( -3.999999999999998224, -1.656854249492383024, 11.18750000273119660 ) ) ;
#4176=CYLINDRICAL_SURFACE ( 'NONE', #3357, 4.000000000000000000 ) ;
#4184=CARTESIAN_POINT ( 'NONE',  ( -3.999999999999999112, 0.000000000000000000, 13.00000000000001066 ) ) ;
#4194=CARTESIAN_POINT ( 'NONE',  ( -27.50000000000000711, 7.500000000000002665, -33.66025403784446723 ) ) ;
#4196=CARTESIAN_POINT ( 'NONE',  ( 2.445694354108821411, 2.445694354108820523, 15.06250000136560452 ) ) ;
#4202=CARTESIAN_POINT ( 'NONE',  ( -2.445694354108818303, -2.445694354108820523, 11.56250000136560629 ) ) ;
#4207=ORIENTED_EDGE ( 'NONE', *, *, #6324, .T. ) ;
#4216=ORIENTED_EDGE ( 'NONE', *, *, #9504, .T. ) ;
#4217=CARTESIAN_POINT ( 'NONE',  ( 3.458734125000001658, 1.432654583217640498, 16.25000000136560629 ) ) ;
#4229=CARTESIAN_POINT ( 'NONE',  ( -1.432654583217638944, 3.458734125000000326, 10.25000000136560629 ) ) ;
#4230=CARTESIAN_POINT ( 'NONE',  ( -1.656854249492379250, 4.000000000000000000, 16.93750000273119838 ) ) ;
#4239=CIRCLE ( 'NONE', #21818, 4.000000000000000000 ) ;
#4244=CARTESIAN_POINT ( 'NONE',  ( 4.000000000000000888, 4.898587196589412829E-16, 14.50000000000001066 ) ) ;
#4248=EDGE_CURVE ( 'NONE', #19691, #14136, #6401, .T. ) ;
#4259=CARTESIAN_POINT ( 'NONE',  ( -2.445694354108819191, 2.445694354108820523, 15.56250000136560629 ) ) ;
#4269=ORIENTED_EDGE ( 'NONE', *, *, #19420, .T. ) ;
#4278=CARTESIAN_POINT ( 'NONE',  ( 2.828427124746192067, -2.828427124746189847, 19.37500000000001066 ) ) ;
#4285=CARTESIAN_POINT ( 'NONE',  ( 2.445694354108821411, 2.445694354108820523, 18.06250000136560274 ) ) ;
#4295=CARTESIAN_POINT ( 'NONE',  ( 9.920644283265380691E-16, 4.000000000000000000, 14.87500000273119660 ) ) ;
#4299=CARTESIAN_POINT ( 'NONE',  ( -0.3649867057748917842, 3.983313282257320509, 9.889028792932920808 ) ) ;
#4304=CARTESIAN_POINT ( 'NONE',  ( 4.000000000000001776, -1.656854249492379694, 13.43750000000001243 ) ) ;
#4311=DIRECTION ( 'NONE',  ( -0.000000000000000000, 1.000000000000000000, -0.000000000000000000 ) ) ;
#4313=CARTESIAN_POINT ( 'NONE',  ( -3.458734124999998993, 1.432654583217640276, 15.37500000136560807 ) ) ;
#4315=LINE ( 'NONE', #13674, #2707 ) ;
#4330=CARTESIAN_POINT ( 'NONE',  ( -2.445694354108819191, 2.445694354108820523, 17.56250000136560274 ) ) ;
#4342=CARTESIAN_POINT ( 'NONE',  ( 4.000000000000000888, 4.898587196589412829E-16, 13.62500000273119660 ) ) ;
#4346=ORIENTED_EDGE ( 'NONE', *, *, #11430, .F. ) ;
#4347=CARTESIAN_POINT ( 'NONE',  ( -2.762848947613220307, 4.746226468750993632, 10.00000000000000888 ) ) ;
#4354=CARTESIAN_POINT ( 'NONE',  ( -3.999999999999999112, 0.000000000000000000, 12.00000000000001066 ) ) ;
#4363=CARTESIAN_POINT ( 'NONE',  ( 1.432654583217643163, -3.458734124999999882, 18.00000000136560274 ) ) ;
#4370=CARTESIAN_POINT ( 'NONE',  ( 3.458734125000002546, -1.432654583217639610, 12.12500000136560629 ) ) ;
#4375=CARTESIAN_POINT ( 'NONE',  ( 14.99999999999999645, 10.00000000000000000, -20.00000000000000355 ) ) ;
#4397=CARTESIAN_POINT ( 'NONE',  ( -3.999999999999999112, 0.000000000000000000, 12.12500000273119838 ) ) ;
#4400=LINE ( 'NONE', #16749, #21963 ) ;
#4414=ORIENTED_EDGE ( 'NONE', *, *, #21485, .T. ) ;
#4417=CARTESIAN_POINT ( 'NONE',  ( 14.99999999999995559, 15.00000000000000000, -50.00000000000000000 ) ) ;
#4418=DIRECTION ( 'NONE',  ( -1.224646799147353207E-16, 0.000000000000000000, -1.000000000000000000 ) ) ;
#4420=VERTEX_POINT ( 'NONE', #10473 ) ;
#4421=CARTESIAN_POINT ( 'NONE',  ( 35.00000000000000000, 4.500000000000001776, -20.00000000000000355 ) ) ;
#4424=ORIENTED_EDGE ( 'NONE', *, *, #19916, .T. ) ;
#4428=CARTESIAN_POINT ( 'NONE',  ( 2.828427124746192067, -2.828427124746189847, 10.50000000273119660 ) ) ;
#4431=CARTESIAN_POINT ( 'NONE',  ( 1.432654583217641164, 3.458734125000000326, 15.12500000136560807 ) ) ;
#4449=CARTESIAN_POINT ( 'NONE',  ( 3.458734125000001658, 4.235727675282972223E-16, 17.18750000136560629 ) ) ;
#4459=CARTESIAN_POINT ( 'NONE',  ( 1.971781867644420635E-15, -4.000000000000000000, 10.37500000273119660 ) ) ;
#4462=CARTESIAN_POINT ( 'NONE',  ( 9.920644283265380691E-16, 4.000000000000000000, 13.75000000000001066 ) ) ;
#4469=CARTESIAN_POINT ( 'NONE',  ( 1.971781867644420635E-15, -4.000000000000000000, 14.25000000000001066 ) ) ;
#4471=CARTESIAN_POINT ( 'NONE',  ( 14.99999999999995914, 15.00000000000000000, -20.00000000000000355 ) ) ;
#4477=DIRECTION ( 'NONE',  ( -1.000000000000000000, 0.000000000000000000, 0.000000000000000000 ) ) ;
#4482=VECTOR ( 'NONE', #19311, 1000.000000000000114 ) ;
#4486=CARTESIAN_POINT ( 'NONE',  ( 1.025207404391860050E-15, 3.458734125000000770, 10.43750000136560629 ) ) ;
#4493=( LENGTH_UNIT ( ) NAMED_UNIT ( * ) SI_UNIT ( .MILLI., .METRE. ) );
#4495=VERTEX_POINT ( 'NONE', #10234 ) ;
#4507=EDGE_CURVE ( 'NONE', #18318, #10729, #6739, .T. ) ;
#4513=CARTESIAN_POINT ( 'NONE',  ( 1.236993788156008760E-15, 0.000000000000000000, 21.31370849898476649 ) ) ;
#4516=CARTESIAN_POINT ( 'NONE',  ( 3.458734125000002102, -1.432654583217639610, 17.87500000136560274 ) ) ;
#4524=CARTESIAN_POINT ( 'NONE',  ( -1.656854249492380138, -3.999999999999999112, 12.18750000000001066 ) ) ;
#4526=VERTEX_POINT ( 'NONE', #4934 ) ;
#4539=EDGE_CURVE ( 'NONE', #17227, #22113, #4017, .T. ) ;
#4542=CARTESIAN_POINT ( 'NONE',  ( 1.656854249492384135, -3.999999999999999112, 19.31250000000001421 ) ) ;
#4548=LINE ( 'NONE', #17370, #2622 ) ;
#4550=CARTESIAN_POINT ( 'NONE',  ( -2.445694354108819191, 2.445694354108820523, 15.31250000136560452 ) ) ;
#4553=CARTESIAN_POINT ( 'NONE',  ( -14.99999999999997335, 15.00000000000000000, -49.99999999999999289 ) ) ;
#4563=ORIENTED_EDGE ( 'NONE', *, *, #8664, .T. ) ;
#4571=EDGE_CURVE ( 'NONE', #17488, #2257, #10596, .T. ) ;
#4573=CARTESIAN_POINT ( 'NONE',  ( 1.432654583217641386, 3.458734125000000770, 14.37500000136560452 ) ) ;
#4578=FACE_BOUND ( 'NONE', #10840, .T. ) ;
#4585=CARTESIAN_POINT ( 'NONE',  ( 2.828427124746191179, 2.828427124746190291, 10.75000000273119660 ) ) ;
#4590=CARTESIAN_POINT ( 'NONE',  ( -1.656854249492379472, 4.000000000000000000, 16.93750000273119838 ) ) ;
#4595=EDGE_LOOP ( 'NONE', ( #9732, #17463, #21178, #272 ) ) ;
#4608=CARTESIAN_POINT ( 'NONE',  ( -3.458734124999999437, 0.000000000000000000, 18.68750000136560629 ) ) ;
#4609=CARTESIAN_POINT ( 'NONE',  ( 9.920644283265380691E-16, 4.000000000000000000, 11.87500000273119660 ) ) ;
#4617=CARTESIAN_POINT ( 'NONE',  ( 3.458734125000002546, -1.432654583217639610, 11.12500000136560452 ) ) ;
#4651=CARTESIAN_POINT ( 'NONE',  ( -2.247776618166720475, 3.308700692843488333, 9.970592379354943802 ) ) ;
#4655=CARTESIAN_POINT ( 'NONE',  ( 1.656854249492381470, 4.000000000000000000, 17.68750000000001066 ) ) ;
#4657=CARTESIAN_POINT ( 'NONE',  ( 1.971781867644420635E-15, -4.000000000000000000, 16.25000000000001066 ) ) ;
#4658=CARTESIAN_POINT ( 'NONE',  ( -14.99999999999997335, 15.00000000000000000, -49.99999999999999289 ) ) ;
#4664=CARTESIAN_POINT ( 'NONE',  ( 1.656854249492384135, -3.999999999999999112, 10.43750000273119660 ) ) ;
#4666=CARTESIAN_POINT ( 'NONE',  ( 3.458734125000002102, -1.432654583217639610, 12.87500000136560629 ) ) ;
#4670=CARTESIAN_POINT ( 'NONE',  ( -1.656854249492379472, 4.000000000000000000, 15.81250000000001066 ) ) ;
#4684=CARTESIAN_POINT ( 'NONE',  ( -1.432654583217639832, -3.458734125000000326, 13.87500000136560452 ) ) ;
#4699=CARTESIAN_POINT ( 'NONE',  ( -3.999999999999999112, 1.656854249492380804, 12.06250000273119838 ) ) ;
#4700=DIRECTION ( 'NONE',  ( 0.9413949561959078505, 0.3373062947069098150, 0.000000000000000000 ) ) ;
#4711=CIRCLE ( 'NONE', #13910, 2.649999999999992806 ) ;
#4713=ORIENTED_EDGE ( 'NONE', *, *, #2592, .T. ) ;
#4718=CARTESIAN_POINT ( 'NONE',  ( -0.3649867057748917842, 3.983313282257320509, 9.889028792932920808 ) ) ;
#4720=CARTESIAN_POINT ( 'NONE',  ( 1.872352939448454495E-15, -3.458734125000000770, 18.93750000136560629 ) ) ;
#4721=CARTESIAN_POINT ( 'NONE',  ( 1.971781867644420635E-15, -4.000000000000000000, 14.37500000273119660 ) ) ;
#4727=AXIS2_PLACEMENT_3D ( 'NONE', #12245, #19513, #3110 ) ;
#4729=CARTESIAN_POINT ( 'NONE',  ( 1.872352939448454495E-15, -3.458734125000000770, 10.93750000136560452 ) ) ;
#4730=EDGE_CURVE ( 'NONE', #13130, #3140, #4852, .T. ) ;
#4734=ORIENTED_EDGE ( 'NONE', *, *, #19346, .T. ) ;
#4737=ORIENTED_EDGE ( 'NONE', *, *, #3105, .T. ) ;
#4752=CARTESIAN_POINT ( 'NONE',  ( 3.458734125000002102, -1.432654583217639610, 13.87500000136560452 ) ) ;
#4764=VERTEX_POINT ( 'NONE', #16663 ) ;
#4778=CARTESIAN_POINT ( 'NONE',  ( -1.432654583217639610, -3.458734124999999882, 10.62500000136560274 ) ) ;
#4788=ORIENTED_EDGE ( 'NONE', *, *, #13087, .T. ) ;
#4795=ORIENTED_EDGE ( 'NONE', *, *, #4571, .T. ) ;
#4798=ORIENTED_EDGE ( 'NONE', *, *, #22573, .T. ) ;
#4799=CARTESIAN_POINT ( 'NONE',  ( 1.432654583217641386, 3.458734125000000770, 12.37500000136560629 ) ) ;
#4811=CARTESIAN_POINT ( 'NONE',  ( -3.999999999999999112, 0.000000000000000000, 13.00000000000001066 ) ) ;
#4813=CARTESIAN_POINT ( 'NONE',  ( -2.828427124746188515, -2.828427124746190735, 13.25000000273119660 ) ) ;
#4815=ORIENTED_EDGE ( 'NONE', *, *, #20190, .F. ) ;
#4834=CARTESIAN_POINT ( 'NONE',  ( -2.445694354108819191, 2.445694354108820523, 16.56250000136560629 ) ) ;
#4835=CARTESIAN_POINT ( 'NONE',  ( 1.656854249492381470, 4.000000000000000000, 12.81250000273119660 ) ) ;
#4848=CARTESIAN_POINT ( 'NONE',  ( -3.999999999999999112, 0.000000000000000000, 15.12500000273119660 ) ) ;
#4852=( BOUNDED_CURVE ( )  B_SPLINE_CURVE ( 2, ( #124, #598, #7924, #7455, #9485, #5998, #16785, #2281, #14770 ),
 .UNSPECIFIED., .F., .F. ) 
 B_SPLINE_CURVE_WITH_KNOTS ( ( 3, 2, 2, 2, 3 ),
 ( 0.6999999999999999556, 0.7125000000000000222, 0.7249999999999999778, 0.7375000000000000444, 0.7500000000000000000 ),
 .UNSPECIFIED. ) 
 CURVE ( )  GEOMETRIC_REPRESENTATION_ITEM ( )  RATIONAL_B_SPLINE_CURVE ( ( 1.000000000000000000, 0.9238795325112867385, 1.000000000000000000, 0.9238795325112867385, 1.000000000000000000, 0.9238795325112867385, 1.000000000000000000, 0.9238795325112867385, 1.000000000000000000 ) ) 
 REPRESENTATION_ITEM ( '' )  );
#4860=EDGE_CURVE ( 'NONE', #1132, #17303, #16196, .T. ) ;
#4870=CARTESIAN_POINT ( 'NONE',  ( 2.445694354108821855, -2.445694354108820079, 13.81250000136560629 ) ) ;
#4878=AXIS2_PLACEMENT_3D ( 'NONE', #20060, #5589, #20180 ) ;
#4892=VECTOR ( 'NONE', #15943, 1000.000000000000000 ) ;
#4902=CARTESIAN_POINT ( 'NONE',  ( -3.458734124999999437, 1.432654583217640498, 18.62500000136560274 ) ) ;
#4912=CARTESIAN_POINT ( 'NONE',  ( -3.999999999999999112, 0.000000000000000000, 13.12500000273119660 ) ) ;
#4914=LINE ( 'NONE', #10691, #5536 ) ;
#4920=CARTESIAN_POINT ( 'NONE',  ( -1.432654583217639166, 3.458734125000000770, 12.50000000136560452 ) ) ;
#4931=VECTOR ( 'NONE', #14871, 1000.000000000000000 ) ;
#4933=CARTESIAN_POINT ( 'NONE',  ( 1.656854249492384135, -3.999999999999999112, 13.31250000000001243 ) ) ;
#4934=CARTESIAN_POINT ( 'NONE',  ( 27.50000000000000000, 7.500000000000002665, -36.31025403784445160 ) ) ;
#4935=CARTESIAN_POINT ( 'NONE',  ( -1.656854249492379250, 4.000000000000000000, 9.937500002731198379 ) ) ;
#4938=LINE ( 'NONE', #13946, #2073 ) ;
#4943=AXIS2_PLACEMENT_3D ( 'NONE', #2144, #10, #16778 ) ;
#4949=VERTEX_POINT ( 'NONE', #2860 ) ;
#4958=( BOUNDED_CURVE ( )  B_SPLINE_CURVE ( 2, ( #823, #6466, #17605, #4542, #19370, #1170, #22737, #6348, #10436 ),
 .UNSPECIFIED., .F., .F. ) 
 B_SPLINE_CURVE_WITH_KNOTS ( ( 3, 2, 2, 2, 3 ),
 ( 0.05000000000000000278, 0.06250000000000000000, 0.07499999999999999722, 0.08749999999999999445, 0.1000000000000000056 ),
 .UNSPECIFIED. ) 
 CURVE ( )  GEOMETRIC_REPRESENTATION_ITEM ( )  RATIONAL_B_SPLINE_CURVE ( ( 1.000000000000000000, 0.9238795325112867385, 1.000000000000000000, 0.9238795325112867385, 1.000000000000000000, 0.9238795325112867385, 1.000000000000000000, 0.9238795325112867385, 1.000000000000000000 ) ) 
 REPRESENTATION_ITEM ( '' )  );
#4959=CARTESIAN_POINT ( 'NONE',  ( -1.432654583217639166, 3.458734125000000770, 14.50000000136560629 ) ) ;
#4998=CARTESIAN_POINT ( 'NONE',  ( -3.458734124999998105, 1.432654583217640276, 15.37500000136560807 ) ) ;
#5004=DIRECTION ( 'NONE',  ( 0.000000000000000000, 0.000000000000000000, 1.000000000000000000 ) ) ;
#5013=ORIENTED_EDGE ( 'NONE', *, *, #21248, .F. ) ;
#5024=CARTESIAN_POINT ( 'NONE',  ( -3.458734124999999437, 0.000000000000000000, 18.68750000136560629 ) ) ;
#5026=CARTESIAN_POINT ( 'NONE',  ( 14.99999999999995914, -15.00000000000000000, -20.00000000000000355 ) ) ;
#5032=ORIENTED_EDGE ( 'NONE', *, *, #15085, .F. ) ;
#5041=CARTESIAN_POINT ( 'NONE',  ( -3.458734124999998993, -1.432654583217642497, 14.75000000136560452 ) ) ;
#5051=CARTESIAN_POINT ( 'NONE',  ( -2.445694354108818303, -2.445694354108820523, 18.56250000136560629 ) ) ;
#5055=ORIENTED_EDGE ( 'NONE', *, *, #20495, .T. ) ;
#5061=CARTESIAN_POINT ( 'NONE',  ( 1.236993788156008760E-15, 0.000000000000000000, 21.31370849898476649 ) ) ;
#5067=EDGE_CURVE ( 'NONE', #3140, #18283, #2259, .T. ) ;
#5069=LINE ( 'NONE', #12402, #18256 ) ;
#5071=CARTESIAN_POINT ( 'NONE',  ( 2.445694354108822299, -2.445694354108820079, 16.06250000136560629 ) ) ;
#5072=CARTESIAN_POINT ( 'NONE',  ( -1.656854249492379250, 4.000000000000000000, 10.93750000273119483 ) ) ;
#5079=EDGE_LOOP ( 'NONE', ( #8233, #613, #14087, #10915, #5013, #4139, #13147, #21089, #12455, #13370, #19073, #20361, #15781, #17713, #21440, #9630 ) ) ;
#5080=DIRECTION ( 'NONE',  ( 0.000000000000000000, 0.000000000000000000, 1.000000000000000000 ) ) ;
#5094=( BOUNDED_CURVE ( )  B_SPLINE_CURVE ( 2, ( #10139, #21105, #13496, #11819, #12053, #19093, #13727, #20989, #11587, #20756, #15648, #6647, #4720, #6409, #15416, #644, #4608, #19209, #19319, #17431, #9901, #18970, #8328, #2908, #10255, #17548, #772, #4363, #11700, #2686, #10027, #1112, #8458, #15765, #13960, #17889, #19791, #21458, #10494, #18013, #7120, #21699, #12165, #19555, #14316, #16219, #8926, #12292, #23631, #3513, #4834, #19669, #10736, #14433, #16108, #1588, #19436, #21575, #5071, #3274, #23506, #23147, #1346, #10381, #8682, #23392, #3391, #15873, #21219, #1466, #15983, #6759, #21339, #23271, #3033, #17666, #17775, #5310, #12650, #10617, #12404, #7244, #14075, #4959, #3150, #18122, #1701, #1227, #8810, #14199, #6996, #6878, #8565, #5188, #12529, #19910, #10846, #9045, #16335, #7364, #5427, #20258, #16809, #257, #16565, #18360, #22041, #9168, #2174, #34, #7477, #3979, #12764, #11316, #1941, #20128, #3863, #3734, #20016, #9280, #18472, #18591, #389, #7720, #12873, #9511, #5659, #7591, #12994, #15033, #16455, #14913, #22290, #22171, #14672, #14560, #21933, #5541, #5785, #21824, #1818, #3618, #11198, #2050, #11074, #9392, #16686, #13114, #10958 ),
 .UNSPECIFIED., .F., .F. ) 
 B_SPLINE_CURVE_WITH_KNOTS ( ( 3, 2, 2, 2, 2, 2, 2, 2, 2, 2, 2, 2, 2, 2, 2, 2, 2, 2, 2, 2, 2, 2, 2, 2, 2, 2, 2, 2, 2, 2, 2, 2, 2, 2, 2, 2, 2, 2, 2, 2, 2, 2, 2, 2, 2, 2, 2, 2, 2, 2, 2, 2, 2, 2, 2, 2, 2, 2, 2, 2, 2, 2, 2, 2, 2, 2, 2, 2, 2, 2, 2, 2, 2, 2, 3 ),
 ( 0.000000000000000000, 0.01250000000000000069, 0.02500000000000000139, 0.03749999999999999861, 0.05000000000000000278, 0.06250000000000000000, 0.07499999999999999722, 0.08749999999999999445, 0.1000000000000000056, 0.1125000000000000028, 0.1250000000000000000, 0.1375000000000000111, 0.1499999999999999944, 0.1625000000000000056, 0.1749999999999999889, 0.1875000000000000278, 0.2000000000000000111, 0.2124999999999999944, 0.2250000000000000056, 0.2374999999999999889, 0.2500000000000000000, 0.2625000000000000111, 0.2750000000000000222, 0.2874999999999999778, 0.2999999999999999889, 0.3125000000000000000, 0.3250000000000000111, 0.3375000000000000777, 0.3499999999999999778, 0.3624999999999999889, 0.3750000000000000555, 0.3875000000000000111, 0.4000000000000000222, 0.4124999999999999223, 0.4249999999999999889, 0.4375000000000000000, 0.4500000000000000111, 0.4625000000000000222, 0.4749999999999999778, 0.4874999999999999889, 0.5000000000000000000, 0.5124999999999999556, 0.5250000000000000222, 0.5374999999999999778, 0.5500000000000000444, 0.5625000000000000000, 0.5749999999999999556, 0.5875000000000000222, 0.5999999999999999778, 0.6125000000000000444, 0.6250000000000000000, 0.6374999999999999556, 0.6500000000000000222, 0.6624999999999999778, 0.6750000000000001554, 0.6875000000000000000, 0.6999999999999999556, 0.7125000000000001332, 0.7249999999999999778, 0.7375000000000000444, 0.7500000000000001110, 0.7624999999999999556, 0.7750000000000000222, 0.7874999999999998668, 0.8000000000000000444, 0.8125000000000000000, 0.8249999999999998446, 0.8375000000000000222, 0.8499999999999999778, 0.8625000000000000444, 0.8750000000000000000, 0.8874999999999999556, 0.9000000000000000222, 0.9124999999999999778, 0.9250000000000000444 ),
 .UNSPECIFIED. ) 
 CURVE ( )  GEOMETRIC_REPRESENTATION_ITEM ( )  RATIONAL_B_SPLINE_CURVE ( ( 1.000000000000000000, 0.9238795325112867385, 1.000000000000000000, 0.9238795325112867385, 1.000000000000000000, 0.9238795325112867385, 1.000000000000000000, 0.9238795325112867385, 1.000000000000000000, 0.9238795325112867385, 1.000000000000000000, 0.9238795325112867385, 1.000000000000000000, 0.9238795325112867385, 1.000000000000000000, 0.9238795325112867385, 1.000000000000000000, 0.9238795325112867385, 1.000000000000000000, 0.9238795325112867385, 1.000000000000000000, 0.9238795325112867385, 1.000000000000000000, 0.9238795325112867385, 1.000000000000000000, 0.9238795325112867385, 1.000000000000000000, 0.9238795325112867385, 1.000000000000000000, 0.9238795325112867385, 1.000000000000000000, 0.9238795325112867385, 1.000000000000000000, 0.9238795325112867385, 1.000000000000000000, 0.9238795325112867385, 1.000000000000000000, 0.9238795325112867385, 1.000000000000000000, 0.9238795325112867385, 1.000000000000000000, 0.9238795325112867385, 1.000000000000000000, 0.9238795325112867385, 1.000000000000000000, 0.9238795325112867385, 1.000000000000000000, 0.9238795325112867385, 1.000000000000000000, 0.9238795325112867385, 1.000000000000000000, 0.9238795325112867385, 1.000000000000000000, 0.9238795325112867385, 1.000000000000000000, 0.9238795325112867385, 1.000000000000000000, 0.9238795325112867385, 1.000000000000000000, 0.9238795325112867385, 1.000000000000000000, 0.9238795325112867385, 1.000000000000000000, 0.9238795325112867385, 1.000000000000000000, 0.9238795325112867385, 1.000000000000000000, 0.9238795325112867385, 1.000000000000000000, 0.9238795325112867385, 1.000000000000000000, 0.9238795325112867385, 1.000000000000000000, 0.9238795325112867385, 1.000000000000000000, 0.9238795325112867385, 1.000000000000000000, 0.9238795325112867385, 1.000000000000000000, 0.9238795325112867385, 1.000000000000000000, 0.9238795325112867385, 1.000000000000000000, 0.9238795325112867385, 1.000000000000000000, 0.9238795325112867385, 1.000000000000000000, 0.9238795325112867385, 1.000000000000000000, 0.9238795325112867385, 1.000000000000000000, 0.9238795325112867385, 1.000000000000000000, 0.9238795325112867385, 1.000000000000000000, 0.9238795325112867385, 1.000000000000000000, 0.9238795325112867385, 1.000000000000000000, 0.9238795325112867385, 1.000000000000000000, 0.9238795325112867385, 1.000000000000000000, 0.9238795325112867385, 1.000000000000000000, 0.9238795325112867385, 1.000000000000000000, 0.9238795325112867385, 1.000000000000000000, 0.9238795325112867385, 1.000000000000000000, 0.9238795325112867385, 1.000000000000000000, 0.9238795325112867385, 1.000000000000000000, 0.9238795325112867385, 1.000000000000000000, 0.9238795325112867385, 1.000000000000000000, 0.9238795325112867385, 1.000000000000000000, 0.9238795325112867385, 1.000000000000000000, 0.9238795325112867385, 1.000000000000000000, 0.9238795325112867385, 1.000000000000000000, 0.9238795325112867385, 1.000000000000000000, 0.9238795325112867385, 1.000000000000000000, 0.9238795325112867385, 1.000000000000000000, 0.9238795325112867385, 1.000000000000000000, 0.9238795325112867385, 1.000000000000000000, 0.9238795325112867385, 1.000000000000000000, 0.9238795325112867385, 1.000000000000000000, 0.9238795325112867385, 1.000000000000000000, 0.9238795325112867385, 1.000000000000000000, 0.9238795325112867385, 1.000000000000000000, 0.9238795325112867385, 1.000000000000000000 ) ) 
 REPRESENTATION_ITEM ( '' )  );
#5103=CARTESIAN_POINT ( 'NONE',  ( 19.99999999999998934, 9.999999999999966249, -50.00000000000000000 ) ) ;
#5107=CARTESIAN_POINT ( 'NONE',  ( 2.445694354108821855, -2.445694354108820079, 16.81250000136560629 ) ) ;
#5114=EDGE_LOOP ( 'NONE', ( #16377, #16012, #14760, #10578 ) ) ;
#5135=CARTESIAN_POINT ( 'NONE',  ( 1.872352939448454495E-15, -3.458734125000000770, 17.93750000136560274 ) ) ;
#5152=CARTESIAN_POINT ( 'NONE',  ( 9.920644283265380691E-16, 4.000000000000000000, 19.75000000000001066 ) ) ;
#5166=CARTESIAN_POINT ( 'NONE',  ( -1.027321559264960715, 3.880635692936085679, 9.999401128100736003 ) ) ;
#5167=CARTESIAN_POINT ( 'NONE',  ( 2.445694354108821411, 2.445694354108820523, 17.06250000136560629 ) ) ;
#5171=CARTESIAN_POINT ( 'NONE',  ( -3.999999999999999112, 0.000000000000000000, 14.12500000273119660 ) ) ;
#5188=CARTESIAN_POINT ( 'NONE',  ( -1.432654583217639832, -3.458734125000000326, 13.87500000136560452 ) ) ;
#5195=CARTESIAN_POINT ( 'NONE',  ( 4.000000000000001776, -1.656854249492379694, 18.56250000273119838 ) ) ;
#5206=ORIENTED_EDGE ( 'NONE', *, *, #1894, .F. ) ;
#5207=CARTESIAN_POINT ( 'NONE',  ( 1.971781867644420635E-15, -4.000000000000000000, 15.25000000000001066 ) ) ;
#5212=FACE_OUTER_BOUND ( 'NONE', #10692, .T. ) ;
#5213=CARTESIAN_POINT ( 'NONE',  ( -3.999999999999999112, 0.000000000000000000, 12.00000000000001066 ) ) ;
#5221=CARTESIAN_POINT ( 'NONE',  ( -3.458734124999998105, 1.432654583217640276, 16.37500000136560629 ) ) ;
#5245=CARTESIAN_POINT ( 'NONE',  ( 9.920644283265380691E-16, 4.000000000000000000, 17.87500000273119483 ) ) ;
#5272=CARTESIAN_POINT ( 'NONE',  ( 4.000000000000000888, 4.898587196589412829E-16, 12.62500000273119660 ) ) ;
#5273=CARTESIAN_POINT ( 'NONE',  ( -3.999999999999999112, 0.000000000000000000, 19.00000000000001066 ) ) ;
#5288=CARTESIAN_POINT ( 'NONE',  ( 1.025207404391860050E-15, 3.458734125000000326, 17.18750000136560274 ) ) ;
#5310=CARTESIAN_POINT ( 'NONE',  ( -1.432654583217639832, -3.458734125000000326, 14.87500000136560807 ) ) ;
#5311=CARTESIAN_POINT ( 'NONE',  ( -1.656854249492380138, -3.999999999999999112, 11.31250000273119660 ) ) ;
#5316=CARTESIAN_POINT ( 'NONE',  ( -3.999999999999999112, 0.000000000000000000, 19.12500000273119838 ) ) ;
#5329=CARTESIAN_POINT ( 'NONE',  ( 2.828427124746191179, 2.828427124746190291, 16.62500000000001066 ) ) ;
#5336=DIRECTION ( 'NONE',  ( 1.224646799147353207E-16, -0.000000000000000000, 1.000000000000000000 ) ) ;
#5339=CIRCLE ( 'NONE', #16443, 4.999999999999999112 ) ;
#5358=CARTESIAN_POINT ( 'NONE',  ( -1.656854249492379472, 4.000000000000000000, 13.93750000273119483 ) ) ;
#5371=CARTESIAN_POINT ( 'NONE',  ( 4.000000000000000888, 1.656854249492381248, 17.68750000273119483 ) ) ;
#5374=CARTESIAN_POINT ( 'NONE',  ( -14.99999999999997335, -15.00000000000000000, -49.99999999999999289 ) ) ;
#5391=CARTESIAN_POINT ( 'NONE',  ( 4.000000000000000888, 4.898587196589412829E-16, 21.31370849898476649 ) ) ;
#5393=CARTESIAN_POINT ( 'NONE',  ( 2.828427124746191179, 2.828427124746190291, 18.62500000000001066 ) ) ;
#5394=CARTESIAN_POINT ( 'NONE',  ( -3.458734124999999437, 0.000000000000000000, 10.68750000136560452 ) ) ;
#5405=CARTESIAN_POINT ( 'NONE',  ( -2.445694354108819191, 2.445694354108820523, 19.31250000136560629 ) ) ;
#5409=CARTESIAN_POINT ( 'NONE',  ( -3.458734124999998993, 0.000000000000000000, 19.43750000136560629 ) ) ;
#5418=ORIENTED_EDGE ( 'NONE', *, *, #9504, .F. ) ;
#5421=CARTESIAN_POINT ( 'NONE',  ( 1.432654583217641386, 3.458734125000000770, 19.37500000136560274 ) ) ;
#5427=CARTESIAN_POINT ( 'NONE',  ( 1.025207404391860050E-15, 3.458734125000000770, 13.43750000136560452 ) ) ;
#5446=CARTESIAN_POINT ( 'NONE',  ( -3.999999999999998224, -1.656854249492383246, 19.06250000000001421 ) ) ;
#5473=CARTESIAN_POINT ( 'NONE',  ( -1.656854249492380138, -3.999999999999999112, 18.18750000000001066 ) ) ;
#5475=AXIS2_PLACEMENT_3D ( 'NONE', #18191, #11149, #7068 ) ;
#5484=CARTESIAN_POINT ( 'NONE',  ( 2.828427124746191179, 2.828427124746190291, 18.75000000273119483 ) ) ;
#5498=ORIENTED_EDGE ( 'NONE', *, *, #636, .F. ) ;
#5506=CARTESIAN_POINT ( 'NONE',  ( 1.656854249492381470, 4.000000000000000000, 18.81250000273119483 ) ) ;
#5507=CARTESIAN_POINT ( 'NONE',  ( 1.656854249492381470, 4.000000000000000000, 16.68750000000001066 ) ) ;
#5515=CARTESIAN_POINT ( 'NONE',  ( 3.458734125000001214, 1.432654583217640498, 16.00000000136560629 ) ) ;
#5519=CARTESIAN_POINT ( 'NONE',  ( -2.445694354108818303, -2.445694354108820523, 13.56250000136560629 ) ) ;
#5522=VERTEX_POINT ( 'NONE', #14599 ) ;
#5536=VECTOR ( 'NONE', #1664, 1000.000000000000000 ) ;
#5541=CARTESIAN_POINT ( 'NONE',  ( 3.458734125000002546, -1.432654583217639610, 11.12500000136560452 ) ) ;
#5542=LINE ( 'NONE', #5786, #9583 ) ;
#5547=CARTESIAN_POINT ( 'NONE',  ( 9.920644283265380691E-16, 4.000000000000000000, 15.87500000273119660 ) ) ;
#5553=ORIENTED_EDGE ( 'NONE', *, *, #9100, .F. ) ;
#5561=CARTESIAN_POINT ( 'NONE',  ( 4.000000000000000888, 4.898587196589412829E-16, 15.50000000000001066 ) ) ;
#5564=ORIENTED_EDGE ( 'NONE', *, *, #8393, .F. ) ;
#5568=CARTESIAN_POINT ( 'NONE',  ( 19.99999999999998934, 9.999999999999964473, -50.00000000000000000 ) ) ;
#5577=CARTESIAN_POINT ( 'NONE',  ( 2.445694354108821411, 2.445694354108820523, 17.31250000136560629 ) ) ;
#5586=LINE ( 'NONE', #1749, #10548 ) ;
#5589=DIRECTION ( 'NONE',  ( -1.000000000000000000, 0.000000000000000000, 1.224646799147353207E-16 ) ) ;
#5593=ORIENTED_EDGE ( 'NONE', *, *, #18616, .F. ) ;
#5604=CARTESIAN_POINT ( 'NONE',  ( 1.971781867644420635E-15, -4.000000000000000000, 16.37500000273119838 ) ) ;
#5612=CYLINDRICAL_SURFACE ( 'NONE', #5475, 4.000000000000000000 ) ;
#5622=ORIENTED_EDGE ( 'NONE', *, *, #2592, .F. ) ;
#5623=( BOUNDED_SURFACE ( )  B_SPLINE_SURFACE ( 1, 2, ( 
 ( #5316, #16340, #21581, #19799, #8688, #21707, #18129, #6766, #10746, #5195, #23512, #14082, #21345, #12535, #3397, #18019, #16226, #14439, #12658, #6027, #9285, #5792, #16817, #16691, #7371, #18720, #5666, #16573, #16461, #11080, #18836, #14680, #395, #13356, #2422, #4230, #18366, #22296, #152, #20623, #20133, #264, #9400, #13120, #18477, #21938, #22177, #7602, #40, #1947, #15039, #9644, #5547, #22048, #2181, #14799, #2058, #12880, #11325, #3985, #13236, #14922, #5910, #20264, #12998, #20379, #2311, #4107, #18598, #9520, #3869, #7726, #16935, #3741, #20502, #11447, #511, #7834, #15155, #22416, #11203, #11569, #7482, #17525, #17294, #19189, #2775, #9753, #4342, #21087, #12144, #976, #17051, #10115, #4813, #749, #13831, #17407, #17171, #8305, #10235, #12034, #8436, #22545, #1092, #6153, #8085, #15627, #19297, #11799, #6385, #20738, #22897, #4699, #19411, #20966, #2535, #6511, #626, #7954, #13941, #21199, #11681, #18950, #9876, #2661, #23018, #15395, #22775, #2888, #6623, #8193, #15747, #15274, #4585, #6268, #13476, #22658, #13585, #20852, #4459, #19071, #10003, #13703, #859, #11921, #15507, #4935, #8781 ),
 ( #5409, #17648, #3369, #23610, #12746, #14541, #21312, #8904, #3133, #7223, #6740, #3250, #19649, #23372, #5051, #1209, #16085, #10597, #10358, #12270, #1566, #19892, #8546, #8661, #12509, #1323, #12384, #15853, #21555, #14294, #23486, #17868, #16200, #6852, #15961, #1442, #5288, #14416, #5167, #6976, #23242, #19768, #3493, #23125, #10713, #17990, #7099, #21678, #12632, #10828, #14177, #18103, #1683, #9027, #16320, #21805, #3008, #14047, #19536, #10474, #17755, #21437, #3600, #20352, #15129, #11055, #367, #5769, #3713, #11294, #20473, #22271, #18691, #9147, #4079, #16434, #18342, #2151, #5883, #22025, #16664, #7347, #18568, #15017, #5999, #7573, #12854, #3960, #10939, #22390, #488, #7811, #14654, #21911, #5519, #12974, #9620, #20111, #9374, #9486, #16911, #18455, #16786, #13208, #14892, #16549, #11416, #2282, #1799, #7456, #1922, #19997, #9264, #238, #7700, #22150, #18218, #125, #2033, #14771, #11181, #20239, #16, #5640, #3846, #13096, #4202, #19041, #13560, #20595, #22512, #11895, #6483, #18813, #18927, #22752, #11657, #22636, #2397, #8168, #836, #10090, #6240, #2750, #17143, #2512, #15369, #15601, #950 ) ),
 .UNSPECIFIED., .F., .F., .F. ) 
 B_SPLINE_SURFACE_WITH_KNOTS ( ( 2, 2 ),
 ( 3, 2, 2, 2, 2, 2, 2, 2, 2, 2, 2, 2, 2, 2, 2, 2, 2, 2, 2, 2, 2, 2, 2, 2, 2, 2, 2, 2, 2, 2, 2, 2, 2, 2, 2, 2, 2, 2, 2, 2, 2, 2, 2, 2, 2, 2, 2, 2, 2, 2, 2, 2, 2, 2, 2, 2, 2, 2, 2, 2, 2, 2, 2, 2, 2, 2, 2, 2, 2, 2, 2, 2, 2, 2, 3 ),
 ( 0.000000000000000000, 1.000000000000000000 ),
 ( 0.000000000000000000, 0.01250000000000000069, 0.02500000000000000139, 0.03749999999999999861, 0.05000000000000000278, 0.06250000000000000000, 0.07499999999999999722, 0.08749999999999999445, 0.1000000000000000056, 0.1125000000000000028, 0.1250000000000000000, 0.1375000000000000111, 0.1499999999999999944, 0.1625000000000000056, 0.1749999999999999889, 0.1875000000000000000, 0.2000000000000000111, 0.2124999999999999944, 0.2250000000000000056, 0.2374999999999999889, 0.2500000000000000000, 0.2625000000000000111, 0.2750000000000000222, 0.2874999999999999778, 0.2999999999999999889, 0.3125000000000000000, 0.3250000000000000111, 0.3375000000000000222, 0.3499999999999999778, 0.3624999999999999889, 0.3750000000000000000, 0.3875000000000000111, 0.4000000000000000222, 0.4124999999999999778, 0.4249999999999999889, 0.4375000000000000000, 0.4500000000000000111, 0.4625000000000000222, 0.4749999999999999778, 0.4874999999999999889, 0.5000000000000000000, 0.5124999999999999556, 0.5250000000000000222, 0.5374999999999999778, 0.5500000000000000444, 0.5625000000000000000, 0.5749999999999999556, 0.5875000000000000222, 0.5999999999999999778, 0.6125000000000000444, 0.6250000000000000000, 0.6374999999999999556, 0.6500000000000000222, 0.6624999999999999778, 0.6750000000000000444, 0.6875000000000000000, 0.6999999999999999556, 0.7125000000000000222, 0.7249999999999999778, 0.7375000000000000444, 0.7500000000000000000, 0.7624999999999999556, 0.7750000000000000222, 0.7874999999999999778, 0.8000000000000000444, 0.8125000000000000000, 0.8249999999999999556, 0.8375000000000000222, 0.8499999999999999778, 0.8625000000000000444, 0.8750000000000000000, 0.8874999999999999556, 0.9000000000000000222, 0.9124999999999999778, 0.9250000000000000444 ),
 .UNSPECIFIED. ) 
 GEOMETRIC_REPRESENTATION_ITEM ( )  RATIONAL_B_SPLINE_SURFACE ( (
 ( 1.000000000000000000, 0.9238795325112867385, 1.000000000000000000, 0.9238795325112867385, 1.000000000000000000, 0.9238795325112867385, 1.000000000000000000, 0.9238795325112867385, 1.000000000000000000, 0.9238795325112867385, 1.000000000000000000, 0.9238795325112867385, 1.000000000000000000, 0.9238795325112867385, 1.000000000000000000, 0.9238795325112867385, 1.000000000000000000, 0.9238795325112867385, 1.000000000000000000, 0.9238795325112867385, 1.000000000000000000, 0.9238795325112867385, 1.000000000000000000, 0.9238795325112867385, 1.000000000000000000, 0.9238795325112867385, 1.000000000000000000, 0.9238795325112867385, 1.000000000000000000, 0.9238795325112867385, 1.000000000000000000, 0.9238795325112867385, 1.000000000000000000, 0.9238795325112867385, 1.000000000000000000, 0.9238795325112867385, 1.000000000000000000, 0.9238795325112867385, 1.000000000000000000, 0.9238795325112867385, 1.000000000000000000, 0.9238795325112867385, 1.000000000000000000, 0.9238795325112867385, 1.000000000000000000, 0.9238795325112867385, 1.000000000000000000, 0.9238795325112867385, 1.000000000000000000, 0.9238795325112867385, 1.000000000000000000, 0.9238795325112867385, 1.000000000000000000, 0.9238795325112867385, 1.000000000000000000, 0.9238795325112867385, 1.000000000000000000, 0.9238795325112867385, 1.000000000000000000, 0.9238795325112867385, 1.000000000000000000, 0.9238795325112867385, 1.000000000000000000, 0.9238795325112867385, 1.000000000000000000, 0.9238795325112867385, 1.000000000000000000, 0.9238795325112867385, 1.000000000000000000, 0.9238795325112867385, 1.000000000000000000, 0.9238795325112867385, 1.000000000000000000, 0.9238795325112867385, 1.000000000000000000, 0.9238795325112867385, 1.000000000000000000, 0.9238795325112867385, 1.000000000000000000, 0.9238795325112867385, 1.000000000000000000, 0.9238795325112867385, 1.000000000000000000, 0.9238795325112867385, 1.000000000000000000, 0.9238795325112867385, 1.000000000000000000, 0.9238795325112867385, 1.000000000000000000, 0.9238795325112867385, 1.000000000000000000, 0.9238795325112867385, 1.000000000000000000, 0.9238795325112867385, 1.000000000000000000, 0.9238795325112867385, 1.000000000000000000, 0.9238795325112867385, 1.000000000000000000, 0.9238795325112867385, 1.000000000000000000, 0.9238795325112867385, 1.000000000000000000, 0.9238795325112867385, 1.000000000000000000, 0.9238795325112867385, 1.000000000000000000, 0.9238795325112867385, 1.000000000000000000, 0.9238795325112867385, 1.000000000000000000, 0.9238795325112867385, 1.000000000000000000, 0.9238795325112867385, 1.000000000000000000, 0.9238795325112867385, 1.000000000000000000, 0.9238795325112867385, 1.000000000000000000, 0.9238795325112867385, 1.000000000000000000, 0.9238795325112867385, 1.000000000000000000, 0.9238795325112867385, 1.000000000000000000, 0.9238795325112867385, 1.000000000000000000, 0.9238795325112867385, 1.000000000000000000, 0.9238795325112867385, 1.000000000000000000, 0.9238795325112867385, 1.000000000000000000, 0.9238795325112867385, 1.000000000000000000, 0.9238795325112867385, 1.000000000000000000, 0.9238795325112867385, 1.000000000000000000, 0.9238795325112867385, 1.000000000000000000, 0.9238795325112867385, 1.000000000000000000, 0.9238795325112867385, 1.000000000000000000, 0.9238795325112867385, 1.000000000000000000, 0.9238795325112867385, 1.000000000000000000),
 ( 1.000000000000000000, 0.9238795325112867385, 1.000000000000000000, 0.9238795325112867385, 1.000000000000000000, 0.9238795325112867385, 1.000000000000000000, 0.9238795325112867385, 1.000000000000000000, 0.9238795325112867385, 1.000000000000000000, 0.9238795325112867385, 1.000000000000000000, 0.9238795325112867385, 1.000000000000000000, 0.9238795325112867385, 1.000000000000000000, 0.9238795325112867385, 1.000000000000000000, 0.9238795325112867385, 1.000000000000000000, 0.9238795325112867385, 1.000000000000000000, 0.9238795325112867385, 1.000000000000000000, 0.9238795325112867385, 1.000000000000000000, 0.9238795325112867385, 1.000000000000000000, 0.9238795325112867385, 1.000000000000000000, 0.9238795325112867385, 1.000000000000000000, 0.9238795325112867385, 1.000000000000000000, 0.9238795325112867385, 1.000000000000000000, 0.9238795325112867385, 1.000000000000000000, 0.9238795325112867385, 1.000000000000000000, 0.9238795325112867385, 1.000000000000000000, 0.9238795325112867385, 1.000000000000000000, 0.9238795325112867385, 1.000000000000000000, 0.9238795325112867385, 1.000000000000000000, 0.9238795325112867385, 1.000000000000000000, 0.9238795325112867385, 1.000000000000000000, 0.9238795325112867385, 1.000000000000000000, 0.9238795325112867385, 1.000000000000000000, 0.9238795325112867385, 1.000000000000000000, 0.9238795325112867385, 1.000000000000000000, 0.9238795325112867385, 1.000000000000000000, 0.9238795325112867385, 1.000000000000000000, 0.9238795325112867385, 1.000000000000000000, 0.9238795325112867385, 1.000000000000000000, 0.9238795325112867385, 1.000000000000000000, 0.9238795325112867385, 1.000000000000000000, 0.9238795325112867385, 1.000000000000000000, 0.9238795325112867385, 1.000000000000000000, 0.9238795325112867385, 1.000000000000000000, 0.9238795325112867385, 1.000000000000000000, 0.9238795325112867385, 1.000000000000000000, 0.9238795325112867385, 1.000000000000000000, 0.9238795325112867385, 1.000000000000000000, 0.9238795325112867385, 1.000000000000000000, 0.9238795325112867385, 1.000000000000000000, 0.9238795325112867385, 1.000000000000000000, 0.9238795325112867385, 1.000000000000000000, 0.9238795325112867385, 1.000000000000000000, 0.9238795325112867385, 1.000000000000000000, 0.9238795325112867385, 1.000000000000000000, 0.9238795325112867385, 1.000000000000000000, 0.9238795325112867385, 1.000000000000000000, 0.9238795325112867385, 1.000000000000000000, 0.9238795325112867385, 1.000000000000000000, 0.9238795325112867385, 1.000000000000000000, 0.9238795325112867385, 1.000000000000000000, 0.9238795325112867385, 1.000000000000000000, 0.9238795325112867385, 1.000000000000000000, 0.9238795325112867385, 1.000000000000000000, 0.9238795325112867385, 1.000000000000000000, 0.9238795325112867385, 1.000000000000000000, 0.9238795325112867385, 1.000000000000000000, 0.9238795325112867385, 1.000000000000000000, 0.9238795325112867385, 1.000000000000000000, 0.9238795325112867385, 1.000000000000000000, 0.9238795325112867385, 1.000000000000000000, 0.9238795325112867385, 1.000000000000000000, 0.9238795325112867385, 1.000000000000000000, 0.9238795325112867385, 1.000000000000000000, 0.9238795325112867385, 1.000000000000000000, 0.9238795325112867385, 1.000000000000000000, 0.9238795325112867385, 1.000000000000000000, 0.9238795325112867385, 1.000000000000000000, 0.9238795325112867385, 1.000000000000000000) ) ) 
 REPRESENTATION_ITEM ( '' )  SURFACE ( )  );
#5624=CARTESIAN_POINT ( 'NONE',  ( 9.920644283265380691E-16, 4.000000000000000000, 18.87500000273119838 ) ) ;
#5625=VECTOR ( 'NONE', #16118, 1000.000000000000000 ) ;
#5626=CARTESIAN_POINT ( 'NONE',  ( -3.999999999999999112, 1.656854249492380804, 19.93750000000001066 ) ) ;
#5628=CARTESIAN_POINT ( 'NONE',  ( 9.920644283265380691E-16, 4.000000000000000000, 10.75000000000001066 ) ) ;
#5636=CARTESIAN_POINT ( 'NONE',  ( -3.458734124999998993, 1.432654583217640276, 18.37500000136560274 ) ) ;
#5640=CARTESIAN_POINT ( 'NONE',  ( 1.432654583217643163, -3.458734124999999437, 11.75000000136560629 ) ) ;
#5645=ORIENTED_EDGE ( 'NONE', *, *, #17516, .T. ) ;
#5648=CARTESIAN_POINT ( 'NONE',  ( -3.999999999999998224, -1.656854249492383024, 17.06250000000001066 ) ) ;
#5653=CARTESIAN_POINT ( 'NONE',  ( -2.445694354108819191, 2.445694354108820523, 19.56250000136560629 ) ) ;
#5656=CIRCLE ( 'NONE', #19044, 5.000000000000000888 ) ;
#5659=CARTESIAN_POINT ( 'NONE',  ( -2.445694354108818303, -2.445694354108820967, 11.81250000136560629 ) ) ;
#5666=CARTESIAN_POINT ( 'NONE',  ( 2.828427124746192067, -2.828427124746189847, 17.50000000273119483 ) ) ;
#5669=ORIENTED_EDGE ( 'NONE', *, *, #14272, .T. ) ;
#5670=CARTESIAN_POINT ( 'NONE',  ( 1.236993788156008760E-15, 0.000000000000000000, 21.31370849898476649 ) ) ;
#5677=CARTESIAN_POINT ( 'NONE',  ( 1.656854249492381470, 4.000000000000000000, 15.68750000000001066 ) ) ;
#5689=VECTOR ( 'NONE', #14262, 1000.000000000000000 ) ;
#5690=CARTESIAN_POINT ( 'NONE',  ( 1.236993788156008760E-15, 0.000000000000000000, 21.31370849898476649 ) ) ;
#5695=CARTESIAN_POINT ( 'NONE',  ( -2.445694354108818303, -2.445694354108820967, 14.81250000136560452 ) ) ;
#5702=CARTESIAN_POINT ( 'NONE',  ( -2.828427124746189403, 2.828427124746190291, 12.00000000273119660 ) ) ;
#5706=VERTEX_POINT ( 'NONE', #13426 ) ;
#5712=CARTESIAN_POINT ( 'NONE',  ( 4.000000000000000888, 4.898587196589412829E-16, 18.50000000000001066 ) ) ;
#5713=ORIENTED_EDGE ( 'NONE', *, *, #3228, .F. ) ;
#5722=EDGE_CURVE ( 'NONE', #14480, #16157, #16571, .T. ) ;
#5724=CARTESIAN_POINT ( 'NONE',  ( 2.828427124746191179, 2.828427124746190291, 16.75000000273119838 ) ) ;
#5730=EDGE_CURVE ( 'NONE', #4949, #839, #5743, .T. ) ;
#5736=ORIENTED_EDGE ( 'NONE', *, *, #10708, .T. ) ;
#5737=DIRECTION ( 'NONE',  ( 1.224646799147353207E-16, -0.000000000000000000, 1.000000000000000000 ) ) ;
#5743=LINE ( 'NONE', #18666, #1790 ) ;
#5750=CARTESIAN_POINT ( 'NONE',  ( 1.971781867644420635E-15, -4.000000000000000000, 15.25000000000001066 ) ) ;
#5757=VECTOR ( 'NONE', #6851, 1000.000000000000000 ) ;
#5763=CARTESIAN_POINT ( 'NONE',  ( 1.872352939448454495E-15, -3.458734125000000326, 15.68750000136560629 ) ) ;
#5769=CARTESIAN_POINT ( 'NONE',  ( -1.432654583217638944, 3.458734125000000326, 15.25000000136560807 ) ) ;
#5780=CARTESIAN_POINT ( 'NONE',  ( 2.445694354108822299, -2.445694354108820079, 18.06250000136560274 ) ) ;
#5785=CARTESIAN_POINT ( 'NONE',  ( 2.445694354108822299, -2.445694354108820079, 11.06250000136560452 ) ) ;
#5786=CARTESIAN_POINT ( 'NONE',  ( 14.99999999999995559, 15.00000000000000000, -50.00000000000000000 ) ) ;
#5792=CARTESIAN_POINT ( 'NONE',  ( 1.656854249492381470, 4.000000000000000000, 17.81250000273119483 ) ) ;
#5803=CARTESIAN_POINT ( 'NONE',  ( -3.999999999999999112, 1.656854249492380804, 12.93750000000001243 ) ) ;
#5815=CARTESIAN_POINT ( 'NONE',  ( 1.432654583217643163, -3.458734124999999882, 17.00000000136560629 ) ) ;
#5818=CARTESIAN_POINT ( 'NONE',  ( 4.000000000000000888, 4.898587196589412829E-16, 16.50000000000001066 ) ) ;
#5822=CARTESIAN_POINT ( 'NONE',  ( 4.000000000000000888, 4.898587196589412829E-16, 12.50000000000001066 ) ) ;
#5823=ORIENTED_EDGE ( 'NONE', *, *, #1770, .F. ) ;
#5839=CARTESIAN_POINT ( 'NONE',  ( 1.656854249492381470, 4.000000000000000000, 14.81250000273119483 ) ) ;
#5862=ORIENTED_EDGE ( 'NONE', *, *, #22193, .F. ) ;
#5864=CARTESIAN_POINT ( 'NONE',  ( 1.656854249492384135, -3.999999999999999112, 14.31250000000001066 ) ) ;
#5869=( BOUNDED_CURVE ( )  B_SPLINE_CURVE ( 2, ( #3482, #7336, #7443, #19757, #5628 ),
 .UNSPECIFIED., .F., .F. ) 
 B_SPLINE_CURVE_WITH_KNOTS ( ( 3, 2, 3 ),
 ( 0.9000000000000000222, 0.9124999999999999778, 0.9250000000000000444 ),
 .UNSPECIFIED. ) 
 CURVE ( )  GEOMETRIC_REPRESENTATION_ITEM ( )  RATIONAL_B_SPLINE_CURVE ( ( 1.000000000000000000, 0.9238795325112867385, 1.000000000000000000, 0.9238795325112867385, 1.000000000000000000 ) ) 
 REPRESENTATION_ITEM ( '' )  );
#5878=CARTESIAN_POINT ( 'NONE',  ( 3.458734125000001214, 1.432654583217640498, 19.00000000136560629 ) ) ;
#5883=CARTESIAN_POINT ( 'NONE',  ( -2.445694354108818303, -2.445694354108820523, 14.56250000136560452 ) ) ;
#5897=ORIENTED_EDGE ( 'NONE', *, *, #2134, .T. ) ;
#5898=CARTESIAN_POINT ( 'NONE',  ( 3.458734125000001658, 4.235727675282972223E-16, 16.18750000136560629 ) ) ;
#5910=CARTESIAN_POINT ( 'NONE',  ( -2.828427124746188515, -2.828427124746190735, 15.25000000273119660 ) ) ;
#5918=CARTESIAN_POINT ( 'NONE',  ( 1.025207404391860050E-15, 3.458734125000000326, 10.18750000136560629 ) ) ;
#5920=CARTESIAN_POINT ( 'NONE',  ( 9.920644283265380691E-16, 4.000000000000000000, 13.75000000000001066 ) ) ;
#5937=CARTESIAN_POINT ( 'NONE',  ( -3.458734124999999437, 0.000000000000000000, 16.68750000136560629 ) ) ;
#5941=ORIENTED_EDGE ( 'NONE', *, *, #19677, .F. ) ;
#5942=CARTESIAN_POINT ( 'NONE',  ( 4.000000000000001776, -1.656854249492379694, 14.43750000000001066 ) ) ;
#5956=CARTESIAN_POINT ( 'NONE',  ( -3.999999999999999112, 1.656854249492380804, 19.93750000000001066 ) ) ;
#5959=CARTESIAN_POINT ( 'NONE',  ( -2.828427124746189403, 2.828427124746190291, 13.00000000273119660 ) ) ;
#5962=EDGE_CURVE ( 'NONE', #4764, #22004, #3760, .T. ) ;
#5965=CARTESIAN_POINT ( 'NONE',  ( 0.000000000000000000, 0.000000000000000000, 20.00000000000001066 ) ) ;
#5975=CARTESIAN_POINT ( 'NONE',  ( 2.828427124746191179, 2.828427124746190291, 14.75000000273119660 ) ) ;
#5982=CARTESIAN_POINT ( 'NONE',  ( -1.656854249492380138, -3.999999999999999112, 13.18750000000001243 ) ) ;
#5988=ORIENTED_EDGE ( 'NONE', *, *, #14910, .T. ) ;
#5991=EDGE_CURVE ( 'NONE', #13512, #21587, #14918, .T. ) ;
#5994=CARTESIAN_POINT ( 'NONE',  ( -1.432654583217638944, 3.458734125000000326, 15.25000000136560807 ) ) ;
#5995=CARTESIAN_POINT ( 'NONE',  ( 35.00000000000000000, 4.500000000000001776, -20.00000000000000355 ) ) ;
#5998=CARTESIAN_POINT ( 'NONE',  ( 1.656854249492381470, 4.000000000000000000, 12.68750000000001066 ) ) ;
#5999=CARTESIAN_POINT ( 'NONE',  ( 1.025207404391860050E-15, 3.458734125000000326, 14.18750000136560452 ) ) ;
#6004=CARTESIAN_POINT ( 'NONE',  ( 4.000000000000000888, 4.898587196589412829E-16, 15.62500000273119660 ) ) ;
#6014=CARTESIAN_POINT ( 'NONE',  ( -3.458734124999998993, -1.432654583217642497, 17.75000000136560629 ) ) ;
#6026=CARTESIAN_POINT ( 'NONE',  ( -2.445694354108819191, 2.445694354108820523, 12.31250000136560629 ) ) ;
#6027=CARTESIAN_POINT ( 'NONE',  ( -1.656854249492379250, 4.000000000000000000, 17.93750000273119483 ) ) ;
#6028=CARTESIAN_POINT ( 'NONE',  ( 14.99999999999999289, 10.00000000000000000, -50.00000000000000000 ) ) ;
#6033=CARTESIAN_POINT ( 'NONE',  ( -1.656854249492379472, 4.000000000000000000, 13.81250000000001066 ) ) ;
#6039=CARTESIAN_POINT ( 'NONE',  ( 4.000000000000000888, 4.898587196589412829E-16, 11.50000000000001066 ) ) ;
#6050=CARTESIAN_POINT ( 'NONE',  ( 4.000000000000001776, -1.656854249492379694, 11.43750000000001066 ) ) ;
#6054=CARTESIAN_POINT ( 'NONE',  ( 1.432654583217643163, -3.458734124999999882, 14.00000000136560629 ) ) ;
#6068=EDGE_LOOP ( 'NONE', ( #19811, #18285, #20981, #5564 ) ) ;
#6077=CARTESIAN_POINT ( 'NONE',  ( -2.828427124746189403, 2.828427124746190291, 12.00000000273119660 ) ) ;
#6081=CARTESIAN_POINT ( 'NONE',  ( 3.458734125000002102, -1.432654583217639610, 16.87500000136560629 ) ) ;
#6085=DIRECTION ( 'NONE',  ( 0.3373062947069096484, -0.9413949561959079615, -4.130810741450707148E-17 ) ) ;
#6096=ORIENTED_EDGE ( 'NONE', *, *, #4248, .T. ) ;
#6103=CARTESIAN_POINT ( 'NONE',  ( 4.000000000000000888, 1.656854249492381248, 13.56250000000001066 ) ) ;
#6114=CARTESIAN_POINT ( 'NONE',  ( -35.00000000000000711, 7.500000000000001776, -49.99999999999998579 ) ) ;
#6116=CARTESIAN_POINT ( 'NONE',  ( -1.432654583217639610, -3.458734124999999882, 14.62500000136560629 ) ) ;
#6125=EDGE_LOOP ( 'NONE', ( #17154, #4798, #14221, #5206 ) ) ;
#6132=ORIENTED_EDGE ( 'NONE', *, *, #22768, .F. ) ;
#6140=CARTESIAN_POINT ( 'NONE',  ( 1.872352939448454495E-15, -3.458734125000000770, 15.93750000136560629 ) ) ;
#6144=CIRCLE ( 'NONE', #15719, 2.649999999999989253 ) ;
#6153=CARTESIAN_POINT ( 'NONE',  ( 4.000000000000001776, -1.656854249492379694, 12.56250000273119660 ) ) ;
#6160=VECTOR ( 'NONE', #14149, 1000.000000000000000 ) ;
#6165=CARTESIAN_POINT ( 'NONE',  ( -2.828427124746188515, -2.828427124746190735, 14.12500000000001066 ) ) ;
#6182=CARTESIAN_POINT ( 'NONE',  ( 2.445694354108821411, 2.445694354108820523, 12.31250000136560629 ) ) ;
#6190=ORIENTED_EDGE ( 'NONE', *, *, #13667, .F. ) ;
#6205=CARTESIAN_POINT ( 'NONE',  ( -2.828427124746188515, -2.828427124746190735, 12.25000000273119838 ) ) ;
#6224=CARTESIAN_POINT ( 'NONE',  ( 1.971781867644420635E-15, -4.000000000000000000, 11.25000000000001066 ) ) ;
#6231=PLANE ( 'NONE',  #15673 ) ;
#6233=CARTESIAN_POINT ( 'NONE',  ( -1.432654583217638944, 3.458734125000000326, 12.25000000136560452 ) ) ;
#6240=CARTESIAN_POINT ( 'NONE',  ( -2.445694354108818303, -2.445694354108820523, 10.56250000136560452 ) ) ;
#6252=CARTESIAN_POINT ( 'NONE',  ( -1.432654583217639166, 3.458734125000000770, 16.50000000136560629 ) ) ;
#6268=CARTESIAN_POINT ( 'NONE',  ( 4.000000000000000888, 1.656854249492381248, 10.68750000273119483 ) ) ;
#6281=CARTESIAN_POINT ( 'NONE',  ( -2.828427124746189403, 2.828427124746190291, 13.87500000000001066 ) ) ;
#6293=ADVANCED_FACE ( 'NONE', ( #9679 ), #22092, .F. ) ;
#6298=CARTESIAN_POINT ( 'NONE',  ( -3.458734124999999437, 0.000000000000000000, 11.68750000136560629 ) ) ;
#6324=EDGE_CURVE ( 'NONE', #3286, #10092, #190, .T. ) ;
#6325=DIRECTION ( 'NONE',  ( 0.000000000000000000, 0.000000000000000000, 1.000000000000000000 ) ) ;
#6326=CARTESIAN_POINT ( 'NONE',  ( 3.458734125000001214, 4.235727675282971730E-16, 18.93750000136560629 ) ) ;
#6329=ORIENTED_EDGE ( 'NONE', *, *, #5067, .T. ) ;
#6336=DIRECTION ( 'NONE',  ( -0.000000000000000000, -1.000000000000000000, 0.000000000000000000 ) ) ;
#6341=CARTESIAN_POINT ( 'NONE',  ( 1.236993788156008760E-15, 0.000000000000000000, 21.31370849898476649 ) ) ;
#6345=CARTESIAN_POINT ( 'NONE',  ( 4.000000000000000888, 4.898587196589412829E-16, 17.50000000000001066 ) ) ;
#6348=CARTESIAN_POINT ( 'NONE',  ( -3.999999999999998224, -1.656854249492383024, 19.06250000000001421 ) ) ;
#6357=CARTESIAN_POINT ( 'NONE',  ( 1.872352939448454495E-15, -3.458734125000000326, 14.68750000136560452 ) ) ;
#6375=CARTESIAN_POINT ( 'NONE',  ( 3.458734125000002546, -1.432654583217639610, 14.12500000136560452 ) ) ;
#6385=CARTESIAN_POINT ( 'NONE',  ( -2.828427124746188515, -2.828427124746190735, 12.25000000273119838 ) ) ;
#6398=CARTESIAN_POINT ( 'NONE',  ( 9.920644283265380691E-16, 4.000000000000000000, 19.75000000000001066 ) ) ;
#6401=( BOUNDED_CURVE ( )  B_SPLINE_CURVE ( 2, ( #10056, #15332, #1031, #15684, #19239, #9809, #20793, #562, #6326, #22714, #22830, #11737, #913, #22602, #676, #19000, #21024, #6444, #20903, #803, #9934, #22957, #4285, #8136, #11853, #4516, #19129, #2474, #6565, #22470, #2715, #17346, #7887, #9694, #10176, #13881, #15447, #21139, #18781, #2362, #15206, #6081, #5107, #23547, #19477, #8848, #14238, #12205, #19703, #5221, #7036, #3432, #17585, #12566, #1150, #3075, #10650, #14353, #6792, #1377, #15795, #12439, #6678, #8715, #3307, #4998, #17698, #1509, #10418, #8491, #10531, #19589, #17925, #12327, #13991, #23067, #21253, #14113, #10773, #16258, #1624, #21614, #23311, #1259, #16022, #19825, #3185, #21495, #16143, #4752, #4870, #23429, #7155, #18047, #12088, #8967, #14469, #8598, #19353, #2942, #15904, #23181, #6920, #10295, #21376, #17809, #7833, #15273, #9875, #19945, #20378, #2057, #3544, #12690, #6026, #263, #18719, #20622, #22295, #11324, #18835, #2534, #17170, #16690, #10880, #3984, #15154, #7601, #14920, #11446, #22415, #18949, #20501, #11568, #22544, #16934, #18597, #7953, #625, #18158, #9519, #9752, #2310, #21735, #9399, #2180, #510, #4229, #9643 ),
 .UNSPECIFIED., .F., .F. ) 
 B_SPLINE_CURVE_WITH_KNOTS ( ( 3, 2, 2, 2, 2, 2, 2, 2, 2, 2, 2, 2, 2, 2, 2, 2, 2, 2, 2, 2, 2, 2, 2, 2, 2, 2, 2, 2, 2, 2, 2, 2, 2, 2, 2, 2, 2, 2, 2, 2, 2, 2, 2, 2, 2, 2, 2, 2, 2, 2, 2, 2, 2, 2, 2, 2, 2, 2, 2, 2, 2, 2, 2, 2, 2, 2, 2, 2, 2, 2, 2, 2, 2, 2, 3 ),
 ( 0.000000000000000000, 0.01250000000000000069, 0.02500000000000000139, 0.03749999999999999861, 0.05000000000000000278, 0.06250000000000000000, 0.07499999999999999722, 0.08749999999999999445, 0.1000000000000000056, 0.1125000000000000028, 0.1250000000000000000, 0.1375000000000000111, 0.1499999999999999944, 0.1625000000000000056, 0.1749999999999999889, 0.1875000000000000278, 0.2000000000000000111, 0.2124999999999999944, 0.2250000000000000056, 0.2374999999999999889, 0.2500000000000000000, 0.2625000000000000111, 0.2750000000000000222, 0.2874999999999999778, 0.2999999999999999889, 0.3125000000000000000, 0.3250000000000000111, 0.3375000000000000777, 0.3499999999999999778, 0.3624999999999999889, 0.3750000000000000555, 0.3875000000000000111, 0.4000000000000000222, 0.4124999999999999223, 0.4249999999999999889, 0.4375000000000000000, 0.4500000000000000111, 0.4625000000000000222, 0.4749999999999999778, 0.4874999999999999889, 0.5000000000000000000, 0.5124999999999999556, 0.5250000000000000222, 0.5374999999999999778, 0.5500000000000000444, 0.5625000000000000000, 0.5749999999999999556, 0.5875000000000000222, 0.5999999999999999778, 0.6125000000000000444, 0.6250000000000000000, 0.6374999999999999556, 0.6500000000000000222, 0.6624999999999999778, 0.6750000000000001554, 0.6875000000000000000, 0.6999999999999999556, 0.7125000000000001332, 0.7249999999999999778, 0.7375000000000000444, 0.7500000000000001110, 0.7624999999999999556, 0.7750000000000000222, 0.7874999999999998668, 0.8000000000000000444, 0.8125000000000000000, 0.8249999999999998446, 0.8375000000000000222, 0.8499999999999999778, 0.8625000000000000444, 0.8750000000000000000, 0.8874999999999999556, 0.9000000000000000222, 0.9124999999999999778, 0.9250000000000000444 ),
 .UNSPECIFIED. ) 
 CURVE ( )  GEOMETRIC_REPRESENTATION_ITEM ( )  RATIONAL_B_SPLINE_CURVE ( ( 1.000000000000000000, 0.9238795325112867385, 1.000000000000000000, 0.9238795325112867385, 1.000000000000000000, 0.9238795325112867385, 1.000000000000000000, 0.9238795325112867385, 1.000000000000000000, 0.9238795325112867385, 1.000000000000000000, 0.9238795325112867385, 1.000000000000000000, 0.9238795325112867385, 1.000000000000000000, 0.9238795325112867385, 1.000000000000000000, 0.9238795325112867385, 1.000000000000000000, 0.9238795325112867385, 1.000000000000000000, 0.9238795325112867385, 1.000000000000000000, 0.9238795325112867385, 1.000000000000000000, 0.9238795325112867385, 1.000000000000000000, 0.9238795325112867385, 1.000000000000000000, 0.9238795325112867385, 1.000000000000000000, 0.9238795325112867385, 1.000000000000000000, 0.9238795325112867385, 1.000000000000000000, 0.9238795325112867385, 1.000000000000000000, 0.9238795325112867385, 1.000000000000000000, 0.9238795325112867385, 1.000000000000000000, 0.9238795325112867385, 1.000000000000000000, 0.9238795325112867385, 1.000000000000000000, 0.9238795325112867385, 1.000000000000000000, 0.9238795325112867385, 1.000000000000000000, 0.9238795325112867385, 1.000000000000000000, 0.9238795325112867385, 1.000000000000000000, 0.9238795325112867385, 1.000000000000000000, 0.9238795325112867385, 1.000000000000000000, 0.9238795325112867385, 1.000000000000000000, 0.9238795325112867385, 1.000000000000000000, 0.9238795325112867385, 1.000000000000000000, 0.9238795325112867385, 1.000000000000000000, 0.9238795325112867385, 1.000000000000000000, 0.9238795325112867385, 1.000000000000000000, 0.9238795325112867385, 1.000000000000000000, 0.9238795325112867385, 1.000000000000000000, 0.9238795325112867385, 1.000000000000000000, 0.9238795325112867385, 1.000000000000000000, 0.9238795325112867385, 1.000000000000000000, 0.9238795325112867385, 1.000000000000000000, 0.9238795325112867385, 1.000000000000000000, 0.9238795325112867385, 1.000000000000000000, 0.9238795325112867385, 1.000000000000000000, 0.9238795325112867385, 1.000000000000000000, 0.9238795325112867385, 1.000000000000000000, 0.9238795325112867385, 1.000000000000000000, 0.9238795325112867385, 1.000000000000000000, 0.9238795325112867385, 1.000000000000000000, 0.9238795325112867385, 1.000000000000000000, 0.9238795325112867385, 1.000000000000000000, 0.9238795325112867385, 1.000000000000000000, 0.9238795325112867385, 1.000000000000000000, 0.9238795325112867385, 1.000000000000000000, 0.9238795325112867385, 1.000000000000000000, 0.9238795325112867385, 1.000000000000000000, 0.9238795325112867385, 1.000000000000000000, 0.9238795325112867385, 1.000000000000000000, 0.9238795325112867385, 1.000000000000000000, 0.9238795325112867385, 1.000000000000000000, 0.9238795325112867385, 1.000000000000000000, 0.9238795325112867385, 1.000000000000000000, 0.9238795325112867385, 1.000000000000000000, 0.9238795325112867385, 1.000000000000000000, 0.9238795325112867385, 1.000000000000000000, 0.9238795325112867385, 1.000000000000000000, 0.9238795325112867385, 1.000000000000000000, 0.9238795325112867385, 1.000000000000000000, 0.9238795325112867385, 1.000000000000000000, 0.9238795325112867385, 1.000000000000000000, 0.9238795325112867385, 1.000000000000000000, 0.9238795325112867385, 1.000000000000000000, 0.9238795325112867385, 1.000000000000000000, 0.9238795325112867385, 1.000000000000000000, 0.9238795325112867385, 1.000000000000000000 ) ) 
 REPRESENTATION_ITEM ( '' )  );
#6408=CYLINDRICAL_SURFACE ( 'NONE', #21348, 4.000000000000000000 ) ;
#6409=CARTESIAN_POINT ( 'NONE',  ( -1.432654583217639832, -3.458734125000000326, 18.87500000136560629 ) ) ;
#6418=CARTESIAN_POINT ( 'NONE',  ( -3.458734124999999437, 1.432654583217640498, 12.62500000136560629 ) ) ;
#6422=ORIENTED_EDGE ( 'NONE', *, *, #13492, .F. ) ;
#6444=CARTESIAN_POINT ( 'NONE',  ( -3.458734124999998105, 1.432654583217640276, 18.37500000136560629 ) ) ;
#6446=CIRCLE ( 'NONE', #21703, 4.000000000000000888 ) ;
#6449=LINE ( 'NONE', #15688, #2298 ) ;
#6454=DIRECTION ( 'NONE',  ( -0.000000000000000000, -0.000000000000000000, -1.000000000000000000 ) ) ;
#6466=CARTESIAN_POINT ( 'NONE',  ( 4.000000000000001776, -1.656854249492379694, 19.43750000000001066 ) ) ;
#6470=ADVANCED_FACE ( 'NONE', ( #10280 ), #17333, .F. ) ;
#6476=CARTESIAN_POINT ( 'NONE',  ( 1.025207404391860050E-15, 3.458734125000000326, 13.18750000136560452 ) ) ;
#6483=CARTESIAN_POINT ( 'NONE',  ( 1.025207404391860050E-15, 3.458734125000000326, 11.18750000136560452 ) ) ;
#6495=CARTESIAN_POINT ( 'NONE',  ( 1.025207404391860050E-15, 3.458734125000000770, 13.43750000136560452 ) ) ;
#6496=VECTOR ( 'NONE', #15587, 1000.000000000000000 ) ;
#6507=DIRECTION ( 'NONE',  ( 1.224646799147353207E-16, -0.000000000000000000, 1.000000000000000000 ) ) ;
#6511=CARTESIAN_POINT ( 'NONE',  ( 1.656854249492381470, 4.000000000000000000, 11.81250000273119838 ) ) ;
#6525=CARTESIAN_POINT ( 'NONE',  ( 4.000000000000000888, 4.898587196589412829E-16, 19.50000000000001066 ) ) ;
#6532=CARTESIAN_POINT ( 'NONE',  ( 2.828427124746191179, 2.828427124746190291, 14.75000000273119660 ) ) ;
#6541=CARTESIAN_POINT ( 'NONE',  ( 2.445694354108822299, -2.445694354108820079, 12.06250000136560629 ) ) ;
#6549=CARTESIAN_POINT ( 'NONE',  ( -3.999999999999998224, -1.656854249492383024, 15.18750000273119660 ) ) ;
#6554=CARTESIAN_POINT ( 'NONE',  ( 35.00000000000000000, 4.500000000000001776, -20.00000000000000355 ) ) ;
#6555=ORIENTED_EDGE ( 'NONE', *, *, #18730, .T. ) ;
#6565=CARTESIAN_POINT ( 'NONE',  ( 1.872352939448454495E-15, -3.458734125000000326, 17.68750000136560274 ) ) ;
#6570=DIRECTION ( 'NONE',  ( 0.000000000000000000, -1.000000000000000000, 0.000000000000000000 ) ) ;
#6584=CARTESIAN_POINT ( 'NONE',  ( -2.247776618166720475, 3.308700692843488333, 10.40809237798934994 ) ) ;
#6592=CARTESIAN_POINT ( 'NONE',  ( 2.445694354108822299, -2.445694354108820079, 17.06250000136560629 ) ) ;
#6597=EDGE_CURVE ( 'NONE', #11306, #19691, #23290, .T. ) ;
#6602=CARTESIAN_POINT ( 'NONE',  ( 2.828427124746192067, -2.828427124746189847, 13.50000000273119660 ) ) ;
#6612=CARTESIAN_POINT ( 'NONE',  ( -2.445694354108819191, 2.445694354108820523, 11.56250000136560629 ) ) ;
#6615=FACE_OUTER_BOUND ( 'NONE', #188, .T. ) ;
#6623=CARTESIAN_POINT ( 'NONE',  ( -2.828427124746189403, 2.828427124746190291, 11.00000000273119660 ) ) ;
#6646=( BOUNDED_CURVE ( )  B_SPLINE_CURVE ( 2, ( #3697, #4061, #22010, #2014, #5624, #5506, #22131, #2381, #9711 ),
 .UNSPECIFIED., .F., .F. ) 
 B_SPLINE_CURVE_WITH_KNOTS ( ( 3, 2, 2, 2, 3 ),
 ( 0.000000000000000000, 0.01250000000000000243, 0.02500000000000000486, 0.03749999999999999861, 0.05000000000000000971 ),
 .UNSPECIFIED. ) 
 CURVE ( )  GEOMETRIC_REPRESENTATION_ITEM ( )  RATIONAL_B_SPLINE_CURVE ( ( 1.000000000000000000, 0.9238795325112867385, 1.000000000000000000, 0.9238795325112867385, 1.000000000000000000, 0.9238795325112867385, 1.000000000000000000, 0.9238795325112867385, 1.000000000000000000 ) ) 
 REPRESENTATION_ITEM ( '' )  );
#6647=CARTESIAN_POINT ( 'NONE',  ( 1.432654583217643163, -3.458734124999999882, 19.00000000136560629 ) ) ;
#6648=CARTESIAN_POINT ( 'NONE',  ( 2.828427124746192067, -2.828427124746189847, 14.50000000273119660 ) ) ;
#6662=( NAMED_UNIT ( * ) SI_UNIT ( $, .STERADIAN. ) SOLID_ANGLE_UNIT ( ) );
#6670=CYLINDRICAL_SURFACE ( 'NONE', #23291, 2.649999999999992806 ) ;
#6678=CARTESIAN_POINT ( 'NONE',  ( -2.445694354108818303, -2.445694354108820523, 15.56250000136560629 ) ) ;
#6692=VECTOR ( 'NONE', #8117, 1000.000000000000000 ) ;
#6696=CARTESIAN_POINT ( 'NONE',  ( 4.000000000000001776, -1.656854249492379694, 16.43750000000001066 ) ) ;
#6704=CARTESIAN_POINT ( 'NONE',  ( -3.458734124999999437, 0.000000000000000000, 19.68750000136560629 ) ) ;
#6713=DIRECTION ( 'NONE',  ( 0.000000000000000000, 0.000000000000000000, 1.000000000000000000 ) ) ;
#6723=CARTESIAN_POINT ( 'NONE',  ( 3.458734125000002546, -1.432654583217639610, 11.12500000136560452 ) ) ;
#6726=AXIS2_PLACEMENT_3D ( 'NONE', #10482, #1332, #9629 ) ;
#6730=CARTESIAN_POINT ( 'NONE',  ( 1.236993788156008760E-15, 0.000000000000000000, 21.31370849898476649 ) ) ;
#6739=LINE ( 'NONE', #14046, #21114 ) ;
#6740=CARTESIAN_POINT ( 'NONE',  ( 2.445694354108821855, -2.445694354108820079, 18.81250000136560629 ) ) ;
#6759=CARTESIAN_POINT ( 'NONE',  ( 3.458734125000001658, 1.432654583217640498, 15.25000000136560807 ) ) ;
#6760=CARTESIAN_POINT ( 'NONE',  ( -3.999999999999999112, 1.656854249492380804, 11.06250000273119660 ) ) ;
#6766=CARTESIAN_POINT ( 'NONE',  ( 4.000000000000000888, 1.656854249492381248, 18.68750000273119483 ) ) ;
#6782=EDGE_LOOP ( 'NONE', ( #23335, #12894 ) ) ;
#6792=CARTESIAN_POINT ( 'NONE',  ( 2.445694354108821855, -2.445694354108820079, 15.81250000136560629 ) ) ;
#6816=DIRECTION ( 'NONE',  ( -1.224646799147353207E-16, 0.000000000000000000, -1.000000000000000000 ) ) ;
#6819=CARTESIAN_POINT ( 'NONE',  ( 3.458734125000002546, -1.432654583217639610, 19.12500000136560629 ) ) ;
#6835=CARTESIAN_POINT ( 'NONE',  ( -3.999999999999999112, 1.656854249492380582, 13.06250000273119660 ) ) ;
#6838=CARTESIAN_POINT ( 'NONE',  ( 3.458734125000001658, 4.235727675282972223E-16, 14.18750000136560629 ) ) ;
#6848=( GEOMETRIC_REPRESENTATION_CONTEXT ( 3 ) GLOBAL_UNCERTAINTY_ASSIGNED_CONTEXT ( ( #1138 ) ) GLOBAL_UNIT_ASSIGNED_CONTEXT ( ( #18255, #16590, #19934 ) ) REPRESENTATION_CONTEXT ( 'NONE', 'WORKASPACE' ) );
#6850=CARTESIAN_POINT ( 'NONE',  ( -2.828427124746188515, -2.828427124746190735, 13.12500000000001243 ) ) ;
#6851=DIRECTION ( 'NONE',  ( 0.3373062947069096484, -0.9413949561959079615, -4.130810741450707148E-17 ) ) ;
#6852=CARTESIAN_POINT ( 'NONE',  ( -3.458734124999998993, 1.432654583217640276, 17.37500000136559919 ) ) ;
#6863=VECTOR ( 'NONE', #13438, 1000.000000000000000 ) ;
#6866=DIRECTION ( 'NONE',  ( 1.224646799147353207E-16, -0.000000000000000000, 1.000000000000000000 ) ) ;
#6870=ORIENTED_EDGE ( 'NONE', *, *, #22193, .T. ) ;
#6878=CARTESIAN_POINT ( 'NONE',  ( 1.432654583217643163, -3.458734124999999882, 14.00000000136560452 ) ) ;
#6890=VERTEX_POINT ( 'NONE', #4471 ) ;
#6907=CARTESIAN_POINT ( 'NONE',  ( -2.828427124746189403, 2.828427124746190291, 10.87500000000001066 ) ) ;
#6920=CARTESIAN_POINT ( 'NONE',  ( 2.445694354108821411, 2.445694354108820523, 13.06250000136560452 ) ) ;
#6942=CARTESIAN_POINT ( 'NONE',  ( 1.000350172342868515E-15, 3.864683531250000303, 10.67187500034141046 ) ) ;
#6945=AXIS2_PLACEMENT_3D ( 'NONE', #22238, #7317, #22112 ) ;
#6947=CARTESIAN_POINT ( 'NONE',  ( 35.00000000000000000, 4.500000000000001776, -20.00000000000000355 ) ) ;
#6949=CARTESIAN_POINT ( 'NONE',  ( -1.432654583217639832, -3.458734125000000326, 17.87500000136560274 ) ) ;
#6963=CARTESIAN_POINT ( 'NONE',  ( 9.920644283265380691E-16, 4.000000000000000000, 12.87500000273119660 ) ) ;
#6965=CARTESIAN_POINT ( 'NONE',  ( 1.971781867644420635E-15, -4.000000000000000000, 18.25000000000001066 ) ) ;
#6976=CARTESIAN_POINT ( 'NONE',  ( 3.458734125000001214, 1.432654583217640498, 17.00000000136560629 ) ) ;
#6977=DIRECTION ( 'NONE',  ( -0.8660254037844408170, 0.000000000000000000, 0.4999999999999961697 ) ) ;
#6986=DIRECTION ( 'NONE',  ( -0.000000000000000000, -0.000000000000000000, -1.000000000000000000 ) ) ;
#6996=CARTESIAN_POINT ( 'NONE',  ( 2.445694354108822299, -2.445694354108820079, 14.06250000136560629 ) ) ;
#7005=EDGE_CURVE ( 'NONE', #11553, #5706, #8203, .T. ) ;
#7016=CARTESIAN_POINT ( 'NONE',  ( -2.828427124746188515, -2.828427124746190735, 17.12500000000001066 ) ) ;
#7024=ORIENTED_EDGE ( 'NONE', *, *, #18730, .F. ) ;
#7029=CIRCLE ( 'NONE', #4727, 2.649999999999992806 ) ;
#7036=CARTESIAN_POINT ( 'NONE',  ( -2.445694354108819191, 2.445694354108820523, 16.31250000136560629 ) ) ;
#7037=CARTESIAN_POINT ( 'NONE',  ( -2.828427124746188515, -2.828427124746190735, 18.25000000273119483 ) ) ;
#7040=ORIENTED_EDGE ( 'NONE', *, *, #12050, .F. ) ;
#7044=EDGE_LOOP ( 'NONE', ( #9268, #14051, #19571, #14545 ) ) ;
#7056=ADVANCED_FACE ( 'NONE', ( #12042 ), #1334, .T. ) ;
#7066=LINE ( 'NONE', #23343, #22983 ) ;
#7068=DIRECTION ( 'NONE',  ( -1.000000000000000000, 0.000000000000000000, 0.000000000000000000 ) ) ;
#7072=CARTESIAN_POINT ( 'NONE',  ( 1.236993788156008760E-15, 0.000000000000000000, -20.00000000000000000 ) ) ;
#7076=DIRECTION ( 'NONE',  ( 0.9413949561959079615, 0.3373062947069096484, -0.000000000000000000 ) ) ;
#7077=CIRCLE ( 'NONE', #10154, 2.649999999999989253 ) ;
#7082=CARTESIAN_POINT ( 'NONE',  ( -2.828427124746189403, 2.828427124746190291, 18.87500000000001066 ) ) ;
#7083=CARTESIAN_POINT ( 'NONE',  ( -3.999999999999999112, 1.656854249492380804, 18.93750000000000711 ) ) ;
#7095=LINE ( 'NONE', #2147, #13416 ) ;
#7099=CARTESIAN_POINT ( 'NONE',  ( -2.445694354108818303, -2.445694354108820523, 16.56250000136560629 ) ) ;
#7114=VERTEX_POINT ( 'NONE', #2010 ) ;
#7120=CARTESIAN_POINT ( 'NONE',  ( 3.458734125000001658, 4.235727675282972223E-16, 17.18750000136560629 ) ) ;
#7129=ORIENTED_EDGE ( 'NONE', *, *, #17970, .T. ) ;
#7137=CARTESIAN_POINT ( 'NONE',  ( 1.971781867644420635E-15, -4.000000000000000000, 17.25000000000001066 ) ) ;
#7155=CARTESIAN_POINT ( 'NONE',  ( 1.872352939448454495E-15, -3.458734125000000326, 13.68750000136560629 ) ) ;
#7166=ADVANCED_FACE ( 'NONE', ( #23384 ), #21565, .T. ) ;
#7176=( BOUNDED_CURVE ( )  B_SPLINE_CURVE ( 1, ( #10997, #10779 ),
 .UNSPECIFIED., .F., .F. ) 
 B_SPLINE_CURVE_WITH_KNOTS ( ( 2, 2 ),
 ( 0.000000000000000000, 1.000000000000000000 ),
 .UNSPECIFIED. ) 
 CURVE ( )  GEOMETRIC_REPRESENTATION_ITEM ( )  RATIONAL_B_SPLINE_CURVE ( ( 0.9841097943611589738, 0.9841097943611589738 ) ) 
 REPRESENTATION_ITEM ( '' )  );
#7177=AXIS2_PLACEMENT_3D ( 'NONE', #5670, #10820, #14529 ) ;
#7182=CARTESIAN_POINT ( 'NONE',  ( 4.000000000000001776, -1.656854249492379694, 17.56250000273119838 ) ) ;
#7197=LINE ( 'NONE', #23585, #6160 ) ;
#7208=CARTESIAN_POINT ( 'NONE',  ( 9.920644283265380691E-16, 4.000000000000000000, 16.75000000000001066 ) ) ;
#7215=DIRECTION ( 'NONE',  ( -0.000000000000000000, -0.000000000000000000, -1.000000000000000000 ) ) ;
#7219=CARTESIAN_POINT ( 'NONE',  ( 1.872352939448454495E-15, -3.458734125000000326, 16.68750000136560629 ) ) ;
#7223=CARTESIAN_POINT ( 'NONE',  ( 3.458734125000002102, -1.432654583217639610, 18.87500000136560274 ) ) ;
#7236=CARTESIAN_POINT ( 'NONE',  ( -1.432654583217639166, 3.458734125000000770, 19.50000000136560629 ) ) ;
#7239=EDGE_CURVE ( 'NONE', #21282, #21603, #18873, .T. ) ;
#7244=CARTESIAN_POINT ( 'NONE',  ( -3.458734124999999437, 1.432654583217640498, 14.62500000136560452 ) ) ;
#7251=LINE ( 'NONE', #41, #18735 ) ;
#7252=AXIS2_PLACEMENT_3D ( 'NONE', #12112, #6816, #11883 ) ;
#7263=CARTESIAN_POINT ( 'NONE',  ( -1.656854249492380138, -3.999999999999999112, 18.18750000000001066 ) ) ;
#7264=ORIENTED_EDGE ( 'NONE', *, *, #7667, .T. ) ;
#7269=CARTESIAN_POINT ( 'NONE',  ( 35.00000000000000000, 4.500000000000001776, -20.00000000000000355 ) ) ;
#7283=CARTESIAN_POINT ( 'NONE',  ( 4.000000000000000888, 4.898587196589412829E-16, 18.62500000273119483 ) ) ;
#7286=CARTESIAN_POINT ( 'NONE',  ( 4.000000000000000888, 1.656854249492381248, 11.68750000273119660 ) ) ;
#7289=DIRECTION ( 'NONE',  ( -0.000000000000000000, -0.000000000000000000, -1.000000000000000000 ) ) ;
#7290=ORIENTED_EDGE ( 'NONE', *, *, #21930, .T. ) ;
#7307=VERTEX_POINT ( 'NONE', #11388 ) ;
#7308=CARTESIAN_POINT ( 'NONE',  ( 2.828427124746192067, -2.828427124746189847, 16.50000000273119838 ) ) ;
#7310=CARTESIAN_POINT ( 'NONE',  ( -2.828427124746189403, 2.828427124746190291, 10.00000000273119660 ) ) ;
#7317=DIRECTION ( 'NONE',  ( 1.000000000000000000, 0.000000000000000000, -1.224646799147353207E-16 ) ) ;
#7318=AXIS2_PLACEMENT_3D ( 'NONE', #3111, #10686, #17843 ) ;
#7328=CARTESIAN_POINT ( 'NONE',  ( -27.50000000000000711, 4.500000000000001776, -31.01025403784447221 ) ) ;
#7329=ORIENTED_EDGE ( 'NONE', *, *, #2258, .T. ) ;
#7330=( BOUNDED_CURVE ( )  B_SPLINE_CURVE ( 2, ( #13232, #10961, #20498 ),
 .UNSPECIFIED., .F., .F. ) 
 B_SPLINE_CURVE_WITH_KNOTS ( ( 3, 3 ),
 ( 0.9235200992307018852, 0.9250000000000000444 ),
 .UNSPECIFIED. ) 
 CURVE ( )  GEOMETRIC_REPRESENTATION_ITEM ( )  RATIONAL_B_SPLINE_CURVE ( ( 0.9841097943611589738, 0.9909879409283294249, 1.000000000000000000 ) ) 
 REPRESENTATION_ITEM ( '' )  );
#7332=CARTESIAN_POINT ( 'NONE',  ( 4.000000000000001776, -1.656854249492379694, 17.43750000000001421 ) ) ;
#7334=AXIS2_PLACEMENT_3D ( 'NONE', #17375, #12002, #21168 ) ;
#7336=CARTESIAN_POINT ( 'NONE',  ( -3.999999999999999112, 1.656854249492380582, 10.93750000000001243 ) ) ;
#7343=CARTESIAN_POINT ( 'NONE',  ( -3.458734124999998993, 1.432654583217640276, 19.37500000136560274 ) ) ;
#7347=CARTESIAN_POINT ( 'NONE',  ( -3.458734124999998993, 1.432654583217640276, 14.37500000136560452 ) ) ;
#7349=ADVANCED_FACE ( 'NONE', ( #2377 ), #4176, .T. ) ;
#7364=CARTESIAN_POINT ( 'NONE',  ( -1.432654583217639166, 3.458734125000000770, 13.50000000136560452 ) ) ;
#7371=CARTESIAN_POINT ( 'NONE',  ( 4.000000000000000888, 4.898587196589412829E-16, 17.62500000273119483 ) ) ;
#7378=EDGE_LOOP ( 'NONE', ( #18737, #22846, #14367, #11154 ) ) ;
#7380=( LENGTH_UNIT ( ) NAMED_UNIT ( * ) SI_UNIT ( .MILLI., .METRE. ) );
#7382=LINE ( 'NONE', #13247, #590 ) ;
#7384=CARTESIAN_POINT ( 'NONE',  ( 9.920644283265380691E-16, 4.000000000000000000, 15.75000000000001066 ) ) ;
#7388=CARTESIAN_POINT ( 'NONE',  ( -27.50000000000000711, 7.500000000000002665, -36.31025403784445160 ) ) ;
#7396=CARTESIAN_POINT ( 'NONE',  ( -3.458734124999998993, 1.432654583217640276, 10.37500000136560629 ) ) ;
#7400=CARTESIAN_POINT ( 'NONE',  ( -35.00000000000000000, 7.500000000000001776, -19.99999999999998934 ) ) ;
#7411=CARTESIAN_POINT ( 'NONE',  ( 4.000000000000000888, 4.898587196589412829E-16, 13.62500000273119660 ) ) ;
#7413=AXIS2_PLACEMENT_3D ( 'NONE', #3576, #14386, #22114 ) ;
#7420=CARTESIAN_POINT ( 'NONE',  ( -3.999999999999999112, 1.656854249492380804, 17.06250000273120193 ) ) ;
#7439=EDGE_CURVE ( 'NONE', #7929, #13418, #13869, .T. ) ;
#7440=CARTESIAN_POINT ( 'NONE',  ( -3.999999999999999112, 0.000000000000000000, 15.12500000273119660 ) ) ;
#7441=CARTESIAN_POINT ( 'NONE',  ( -2.828427124746189403, 2.828427124746190291, 19.87500000000001066 ) ) ;
#7443=CARTESIAN_POINT ( 'NONE',  ( -2.828427124746189403, 2.828427124746190291, 10.87500000000001066 ) ) ;
#7451=CARTESIAN_POINT ( 'NONE',  ( -2.445694354108818303, -2.445694354108820523, 16.56250000136560629 ) ) ;
#7455=CARTESIAN_POINT ( 'NONE',  ( -1.656854249492379472, 4.000000000000000000, 12.81250000000001066 ) ) ;
#7456=CARTESIAN_POINT ( 'NONE',  ( -1.432654583217639610, -3.458734124999999882, 12.62500000136560629 ) ) ;
#7463=CARTESIAN_POINT ( 'NONE',  ( 4.000000000000000888, 4.898587196589412829E-16, 21.31370849898476649 ) ) ;
#7468=CARTESIAN_POINT ( 'NONE',  ( 3.458734125000001658, 4.235727675282972223E-16, 19.18750000136560629 ) ) ;
#7477=CARTESIAN_POINT ( 'NONE',  ( -2.445694354108818303, -2.445694354108820967, 12.81250000136560629 ) ) ;
#7482=CARTESIAN_POINT ( 'NONE',  ( -2.828427124746189403, 2.828427124746190291, 14.00000000273119660 ) ) ;
#7494=ORIENTED_EDGE ( 'NONE', *, *, #18616, .T. ) ;
#7495=CARTESIAN_POINT ( 'NONE',  ( 4.000000000000000888, 1.656854249492381248, 16.56250000000001066 ) ) ;
#7511=CARTESIAN_POINT ( 'NONE',  ( -2.445694354108819191, 2.445694354108820523, 16.56250000136560629 ) ) ;
#7516=DIRECTION ( 'NONE',  ( 1.000000000000000000, 0.000000000000000000, 0.000000000000000000 ) ) ;
#7521=CARTESIAN_POINT ( 'NONE',  ( -20.00000000000001066, 4.500000000000001776, -49.99999999999999289 ) ) ;
#7533=CARTESIAN_POINT ( 'NONE',  ( -1.656854249492380138, -3.999999999999999112, 11.18750000000000888 ) ) ;
#7537=CARTESIAN_POINT ( 'NONE',  ( -0.3649867057748841237, 3.983313282257322285, -19.99999999999999289 ) ) ;
#7554=CARTESIAN_POINT ( 'NONE',  ( -3.999999999999999112, 1.656854249492380804, 14.93750000000000888 ) ) ;
#7558=( BOUNDED_CURVE ( )  B_SPLINE_CURVE ( 2, ( #23085, #6696, #15922, #14133, #4657, #11991, #19259, #9223, #23332 ),
 .UNSPECIFIED., .F., .F. ) 
 B_SPLINE_CURVE_WITH_KNOTS ( ( 3, 2, 2, 2, 3 ),
 ( 0.3499999999999999778, 0.3624999999999999889, 0.3750000000000000000, 0.3875000000000000111, 0.4000000000000000222 ),
 .UNSPECIFIED. ) 
 CURVE ( )  GEOMETRIC_REPRESENTATION_ITEM ( )  RATIONAL_B_SPLINE_CURVE ( ( 1.000000000000000000, 0.9238795325112867385, 1.000000000000000000, 0.9238795325112867385, 1.000000000000000000, 0.9238795325112867385, 1.000000000000000000, 0.9238795325112867385, 1.000000000000000000 ) ) 
 REPRESENTATION_ITEM ( '' )  );
#7559=CARTESIAN_POINT ( 'NONE',  ( -3.999999999999999112, 1.656854249492380582, 18.06250000273119483 ) ) ;
#7567=CARTESIAN_POINT ( 'NONE',  ( 1.872352939448454495E-15, -3.458734125000000326, 17.68750000136560274 ) ) ;
#7573=CARTESIAN_POINT ( 'NONE',  ( 1.432654583217641164, 3.458734125000000326, 14.12500000136560452 ) ) ;
#7575=VERTEX_POINT ( 'NONE', #19600 ) ;
#7587=CARTESIAN_POINT ( 'NONE',  ( -2.445694354108818303, -2.445694354108820967, 15.81250000136560629 ) ) ;
#7591=CARTESIAN_POINT ( 'NONE',  ( -3.458734124999998105, -1.432654583217642497, 11.75000000136560629 ) ) ;
#7601=CARTESIAN_POINT ( 'NONE',  ( -3.458734124999998105, -1.432654583217642275, 11.50000000136560452 ) ) ;
#7602=CARTESIAN_POINT ( 'NONE',  ( -3.999999999999998224, -1.656854249492383246, 16.18750000273119838 ) ) ;
#7606=FACE_OUTER_BOUND ( 'NONE', #2102, .T. ) ;
#7613=CARTESIAN_POINT ( 'NONE',  ( -1.656854249492380138, -3.999999999999999112, 13.18750000000001243 ) ) ;
#7630=CARTESIAN_POINT ( 'NONE',  ( 2.445694354108821411, 2.445694354108820523, 13.31250000136560452 ) ) ;
#7639=DIRECTION ( 'NONE',  ( 0.000000000000000000, 0.000000000000000000, 1.000000000000000000 ) ) ;
#7641=ORIENTED_EDGE ( 'NONE', *, *, #17516, .F. ) ;
#7655=CARTESIAN_POINT ( 'NONE',  ( 4.000000000000000888, 4.898587196589412829E-16, 16.62500000273119838 ) ) ;
#7661=DIRECTION ( 'NONE',  ( 0.000000000000000000, 0.000000000000000000, 1.000000000000000000 ) ) ;
#7667=EDGE_CURVE ( 'NONE', #16157, #10374, #11840, .T. ) ;
#7681=CARTESIAN_POINT ( 'NONE',  ( 27.50000000000000000, 7.500000000000001776, -33.66025403784446723 ) ) ;
#7682=ORIENTED_EDGE ( 'NONE', *, *, #17141, .T. ) ;
#7684=CARTESIAN_POINT ( 'NONE',  ( 1.656854249492381470, 4.000000000000000000, 14.68750000000000888 ) ) ;
#7695=CARTESIAN_POINT ( 'NONE',  ( -3.458734124999998993, -1.432654583217642497, 18.50000000136560629 ) ) ;
#7700=CARTESIAN_POINT ( 'NONE',  ( -2.445694354108819191, 2.445694354108820523, 12.31250000136560629 ) ) ;
#7702=ORIENTED_EDGE ( 'NONE', *, *, #13918, .F. ) ;
#7713=CARTESIAN_POINT ( 'NONE',  ( -2.445694354108818303, -2.445694354108820967, 18.81250000136560629 ) ) ;
#7720=CARTESIAN_POINT ( 'NONE',  ( 1.432654583217643163, -3.458734124999999882, 12.00000000136560807 ) ) ;
#7726=CARTESIAN_POINT ( 'NONE',  ( 4.000000000000000888, 1.656854249492381248, 14.68750000273119660 ) ) ;
#7735=ORIENTED_EDGE ( 'NONE', *, *, #20584, .T. ) ;
#7736=CARTESIAN_POINT ( 'NONE',  ( 4.000000000000000888, 1.656854249492381248, 12.56250000000001243 ) ) ;
#7746=LINE ( 'NONE', #22317, #21921 ) ;
#7750=CARTESIAN_POINT ( 'NONE',  ( -3.458734124999999437, 0.000000000000000000, 13.68750000136560629 ) ) ;
#7758=EDGE_LOOP ( 'NONE', ( #11769, #5055, #3857, #11841 ) ) ;
#7772=CARTESIAN_POINT ( 'NONE',  ( -3.999999999999998224, -1.656854249492383246, 13.18750000273119660 ) ) ;
#7773=EDGE_CURVE ( 'NONE', #2992, #14633, #6446, .T. ) ;
#7784=ORIENTED_EDGE ( 'NONE', *, *, #23464, .F. ) ;
#7790=DIRECTION ( 'NONE',  ( -1.000000000000000000, 0.000000000000000000, 0.000000000000000000 ) ) ;
#7796=CARTESIAN_POINT ( 'NONE',  ( 4.000000000000001776, -1.656854249492379694, 15.43750000000001066 ) ) ;
#7800=ORIENTED_EDGE ( 'NONE', *, *, #5730, .T. ) ;
#7806=CARTESIAN_POINT ( 'NONE',  ( -3.458734124999998993, 0.000000000000000000, 15.43750000136560452 ) ) ;
#7811=CARTESIAN_POINT ( 'NONE',  ( 1.432654583217643163, -3.458734124999999437, 13.75000000136560452 ) ) ;
#7813=EDGE_LOOP ( 'NONE', ( #21292, #4207, #9055, #8498 ) ) ;
#7814=CARTESIAN_POINT ( 'NONE',  ( -1.656854249492379472, 4.000000000000000000, 15.93750000273119838 ) ) ;
#7815=VERTEX_POINT ( 'NONE', #21359 ) ;
#7823=CARTESIAN_POINT ( 'NONE',  ( 1.025207404391860050E-15, 3.458734125000000770, 16.43750000136560629 ) ) ;
#7833=CARTESIAN_POINT ( 'NONE',  ( 2.445694354108821855, -2.445694354108820079, 12.81250000136560629 ) ) ;
#7834=CARTESIAN_POINT ( 'NONE',  ( -1.656854249492380138, -3.999999999999999112, 14.31250000273119660 ) ) ;
#7836=ORIENTED_EDGE ( 'NONE', *, *, #9794, .F. ) ;
#7843=CARTESIAN_POINT ( 'NONE',  ( 4.000000000000000888, 1.656854249492381248, 11.56250000000001066 ) ) ;
#7848=VERTEX_POINT ( 'NONE', #6554 ) ;
#7851=CARTESIAN_POINT ( 'NONE',  ( 1.236993788156008760E-15, 0.000000000000000000, 21.31370849898476649 ) ) ;
#7859=CARTESIAN_POINT ( 'NONE',  ( 1.432654583217643163, -3.458734124999999882, 15.00000000136560629 ) ) ;
#7882=CARTESIAN_POINT ( 'NONE',  ( -3.999999999999998224, -1.656854249492383246, 12.18750000273119838 ) ) ;
#7887=CARTESIAN_POINT ( 'NONE',  ( -3.458734124999998993, 0.000000000000000000, 17.43750000136560274 ) ) ;
#7908=CARTESIAN_POINT ( 'NONE',  ( 9.920644283265380691E-16, 4.000000000000000000, 12.75000000000001066 ) ) ;
#7919=CARTESIAN_POINT ( 'NONE',  ( -2.445694354108819191, 2.445694354108820523, 12.31250000136560629 ) ) ;
#7921=DIRECTION ( 'NONE',  ( -1.000000000000000000, 0.000000000000000000, 1.224646799147353207E-16 ) ) ;
#7924=CARTESIAN_POINT ( 'NONE',  ( -2.828427124746189403, 2.828427124746190291, 12.87500000000001066 ) ) ;
#7928=LINE ( 'NONE', #19168, #2844 ) ;
#7929=VERTEX_POINT ( 'NONE', #9064 ) ;
#7939=ORIENTED_EDGE ( 'NONE', *, *, #6324, .F. ) ;
#7940=CARTESIAN_POINT ( 'NONE',  ( -3.458734124999999437, 1.432654583217640498, 17.62500000136560274 ) ) ;
#7943=VECTOR ( 'NONE', #4418, 1000.000000000000000 ) ;
#7953=CARTESIAN_POINT ( 'NONE',  ( 3.458734125000002102, -1.432654583217639610, 10.87500000136560452 ) ) ;
#7954=CARTESIAN_POINT ( 'NONE',  ( 4.000000000000000888, 1.656854249492381248, 11.68750000273119660 ) ) ;
#7965=ORIENTED_EDGE ( 'NONE', *, *, #8208, .T. ) ;
#7966=CARTESIAN_POINT ( 'NONE',  ( 1.656854249492384135, -3.999999999999999112, 11.31250000000001066 ) ) ;
#7970=LINE ( 'NONE', #15170, #2591 ) ;
#7984=CARTESIAN_POINT ( 'NONE',  ( 3.458734125000001658, 4.235727675282972223E-16, 16.18750000136560629 ) ) ;
#8027=CARTESIAN_POINT ( 'NONE',  ( 4.000000000000000888, 4.898587196589412829E-16, 16.62500000273119838 ) ) ;
#8032=STYLED_ITEM ( 'NONE', ( #2820 ), #21929 ) ;
#8033=CARTESIAN_POINT ( 'NONE',  ( -3.999999999999998224, -1.656854249492383246, 15.06250000000001066 ) ) ;
#8034=DIRECTION ( 'NONE',  ( -0.000000000000000000, -0.000000000000000000, -1.000000000000000000 ) ) ;
#8042=ORIENTED_EDGE ( 'NONE', *, *, #12319, .F. ) ;
#8048=CARTESIAN_POINT ( 'NONE',  ( 2.445694354108821855, -2.445694354108820079, 14.81250000136560452 ) ) ;
#8057=EDGE_LOOP ( 'NONE', ( #916, #3703, #14720, #15636 ) ) ;
#8069=CARTESIAN_POINT ( 'NONE',  ( 3.458734125000001658, 1.432654583217640498, 18.25000000136560629 ) ) ;
#8085=CARTESIAN_POINT ( 'NONE',  ( 2.828427124746192067, -2.828427124746189847, 12.50000000273119838 ) ) ;
#8095=CARTESIAN_POINT ( 'NONE',  ( -3.999999999999999112, 1.656854249492380804, 13.93750000000001243 ) ) ;
#8107=CARTESIAN_POINT ( 'NONE',  ( -3.999999999999999112, 0.000000000000000000, 11.00000000000001066 ) ) ;
#8113=CARTESIAN_POINT ( 'NONE',  ( -1.432654583217639832, -3.458734125000000326, 12.87500000136560629 ) ) ;
#8117=DIRECTION ( 'NONE',  ( -1.000000000000000000, 0.000000000000000000, 1.982541115402065110E-16 ) ) ;
#8119=CARTESIAN_POINT ( 'NONE',  ( 4.000000000000000888, 4.898587196589412829E-16, 14.50000000000001066 ) ) ;
#8126=ORIENTED_EDGE ( 'NONE', *, *, #14272, .F. ) ;
#8131=EDGE_CURVE ( 'NONE', #10478, #7307, #13133, .T. ) ;
#8132=ORIENTED_EDGE ( 'NONE', *, *, #14577, .T. ) ;
#8136=CARTESIAN_POINT ( 'NONE',  ( 3.458734125000001214, 1.432654583217640498, 18.00000000136560274 ) ) ;
#8145=CARTESIAN_POINT ( 'NONE',  ( -27.50000000000000711, 7.500000000000002665, -33.66025403784446723 ) ) ;
#8146=CARTESIAN_POINT ( 'NONE',  ( -1.656854249492380138, -3.999999999999999112, 11.31250000273119660 ) ) ;
#8153=CARTESIAN_POINT ( 'NONE',  ( -1.656854249492380138, -3.999999999999999112, 11.18750000000000888 ) ) ;
#8163=CARTESIAN_POINT ( 'NONE',  ( 3.458734125000001214, 4.235727675282971730E-16, 13.93750000136560629 ) ) ;
#8168=CARTESIAN_POINT ( 'NONE',  ( 1.432654583217643163, -3.458734124999999437, 10.75000000136560452 ) ) ;
#8179=CARTESIAN_POINT ( 'NONE',  ( 2.445694354108822299, -2.445694354108820079, 13.06250000136560629 ) ) ;
#8181=CARTESIAN_POINT ( 'NONE',  ( -14.99999999999996980, -15.00000000000000000, -19.99999999999999645 ) ) ;
#8190=( BOUNDED_CURVE ( )  B_SPLINE_CURVE ( 2, ( #11852, #20556, #15331, #19128, #15567, #17345, #6205, #13639, #4397 ),
 .UNSPECIFIED., .F., .F. ) 
 B_SPLINE_CURVE_WITH_KNOTS ( ( 3, 2, 2, 2, 3 ),
 ( 0.6500000000000000222, 0.6624999999999999778, 0.6750000000000000444, 0.6875000000000000000, 0.6999999999999999556 ),
 .UNSPECIFIED. ) 
 CURVE ( )  GEOMETRIC_REPRESENTATION_ITEM ( )  RATIONAL_B_SPLINE_CURVE ( ( 1.000000000000000000, 0.9238795325112867385, 1.000000000000000000, 0.9238795325112867385, 1.000000000000000000, 0.9238795325112867385, 1.000000000000000000, 0.9238795325112867385, 1.000000000000000000 ) ) 
 REPRESENTATION_ITEM ( '' )  );
#8193=CARTESIAN_POINT ( 'NONE',  ( -1.656854249492379250, 4.000000000000000000, 10.93750000273119483 ) ) ;
#8203=LINE ( 'NONE', #12282, #15646 ) ;
#8208=EDGE_CURVE ( 'NONE', #8531, #10374, #19634, .T. ) ;
#8210=EDGE_CURVE ( 'NONE', #8667, #13749, #7970, .T. ) ;
#8218=FACE_OUTER_BOUND ( 'NONE', #6068, .T. ) ;
#8222=CARTESIAN_POINT ( 'NONE',  ( 2.445694354108821411, 2.445694354108820523, 11.31250000136560452 ) ) ;
#8229=AXIS2_PLACEMENT_3D ( 'NONE', #10039, #17326, #891 ) ;
#8233=ORIENTED_EDGE ( 'NONE', *, *, #22573, .F. ) ;
#8252=ORIENTED_EDGE ( 'NONE', *, *, #7005, .F. ) ;
#8260=VECTOR ( 'NONE', #12984, 1000.000000000000000 ) ;
#8271=DIRECTION ( 'NONE',  ( -1.000000000000000000, 0.000000000000000000, 0.000000000000000000 ) ) ;
#8279=CARTESIAN_POINT ( 'NONE',  ( -1.432654583217639610, -3.458734124999999882, 13.62500000136560452 ) ) ;
#8282=ORIENTED_EDGE ( 'NONE', *, *, #15707, .F. ) ;
#8287=ORIENTED_EDGE ( 'NONE', *, *, #3331, .T. ) ;
#8290=ORIENTED_EDGE ( 'NONE', *, *, #1029, .T. ) ;
#8294=CARTESIAN_POINT ( 'NONE',  ( -3.458734124999999437, 1.432654583217640498, 12.62500000136560629 ) ) ;
#8305=CARTESIAN_POINT ( 'NONE',  ( -1.656854249492379250, 4.000000000000000000, 12.93750000273119660 ) ) ;
#8327=( BOUNDED_CURVE ( )  B_SPLINE_CURVE ( 2, ( #10815, #6835, #19521, #16184, #6963, #19633, #10581, #17852, #5272 ),
 .UNSPECIFIED., .F., .F. ) 
 B_SPLINE_CURVE_WITH_KNOTS ( ( 3, 2, 2, 2, 3 ),
 ( 0.5999999999999999778, 0.6125000000000000444, 0.6250000000000000000, 0.6374999999999999556, 0.6500000000000000222 ),
 .UNSPECIFIED. ) 
 CURVE ( )  GEOMETRIC_REPRESENTATION_ITEM ( )  RATIONAL_B_SPLINE_CURVE ( ( 1.000000000000000000, 0.9238795325112867385, 1.000000000000000000, 0.9238795325112867385, 1.000000000000000000, 0.9238795325112867385, 1.000000000000000000, 0.9238795325112867385, 1.000000000000000000 ) ) 
 REPRESENTATION_ITEM ( '' )  );
#8328=CARTESIAN_POINT ( 'NONE',  ( 2.445694354108821411, 2.445694354108820523, 18.31250000136560274 ) ) ;
#8330=CARTESIAN_POINT ( 'NONE',  ( -2.828427124746188515, -2.828427124746190735, 15.25000000273119660 ) ) ;
#8338=CARTESIAN_POINT ( 'NONE',  ( -3.458734124999999437, 0.000000000000000000, 10.68750000136560452 ) ) ;
#8357=EDGE_CURVE ( 'NONE', #1384, #315, #14064, .T. ) ;
#8366=EDGE_CURVE ( 'NONE', #14633, #21075, #824, .T. ) ;
#8393=EDGE_CURVE ( 'NONE', #22113, #19299, #23141, .T. ) ;
#8398=CARTESIAN_POINT ( 'NONE',  ( -1.432654583217639166, 3.458734125000000770, 17.50000000136560274 ) ) ;
#8419=ORIENTED_EDGE ( 'NONE', *, *, #4860, .T. ) ;
#8421=CARTESIAN_POINT ( 'NONE',  ( -3.458734124999998993, -1.432654583217642497, 13.75000000136560452 ) ) ;
#8424=AXIS2_PLACEMENT_3D ( 'NONE', #4513, #9930, #13878 ) ;
#8432=DIRECTION ( 'NONE',  ( -0.000000000000000000, 1.000000000000000000, -0.000000000000000000 ) ) ;
#8436=CARTESIAN_POINT ( 'NONE',  ( 2.828427124746191179, 2.828427124746190291, 12.75000000273119660 ) ) ;
#8437=CARTESIAN_POINT ( 'NONE',  ( -20.00000000000000711, 9.999999999999964473, -19.99999999999999645 ) ) ;
#8458=CARTESIAN_POINT ( 'NONE',  ( -3.458734124999999437, 0.000000000000000000, 17.68750000136560274 ) ) ;
#8459=CARTESIAN_POINT ( 'NONE',  ( 1.656854249492381470, 4.000000000000000000, 13.81250000273119483 ) ) ;
#8467=CARTESIAN_POINT ( 'NONE',  ( -1.432654583217639166, 3.458734125000000770, 12.50000000136560452 ) ) ;
#8487=CARTESIAN_POINT ( 'NONE',  ( 2.828427124746192067, -2.828427124746189847, 17.50000000273119483 ) ) ;
#8488=FACE_OUTER_BOUND ( 'NONE', #9246, .T. ) ;
#8491=CARTESIAN_POINT ( 'NONE',  ( 1.432654583217641164, 3.458734125000000326, 15.12500000136560807 ) ) ;
#8498=ORIENTED_EDGE ( 'NONE', *, *, #8210, .T. ) ;
#8518=CARTESIAN_POINT ( 'NONE',  ( 1.432654583217643163, -3.458734124999999437, 10.75000000136560452 ) ) ;
#8526=EDGE_LOOP ( 'NONE', ( #13437, #21287, #18144, #23383 ) ) ;
#8531=VERTEX_POINT ( 'NONE', #18354 ) ;
#8535=CARTESIAN_POINT ( 'NONE',  ( 2.445694354108821411, 2.445694354108820523, 14.31250000136560452 ) ) ;
#8536=CARTESIAN_POINT ( 'NONE',  ( -35.00000000000000000, 7.500000000000001776, -19.99999999999998934 ) ) ;
#8537=ADVANCED_FACE ( 'NONE', ( #10841 ), #3273, .T. ) ;
#8546=CARTESIAN_POINT ( 'NONE',  ( 2.445694354108821411, 2.445694354108820523, 18.06250000136560274 ) ) ;
#8549=CARTESIAN_POINT ( 'NONE',  ( -2.828427124746188515, -2.828427124746190735, 14.25000000273119660 ) ) ;
#8565=CARTESIAN_POINT ( 'NONE',  ( 1.872352939448454495E-15, -3.458734125000000770, 13.93750000136560629 ) ) ;
#8566=CARTESIAN_POINT ( 'NONE',  ( 4.000000000000000888, 1.656854249492381248, 14.68750000273119660 ) ) ;
#8572=CARTESIAN_POINT ( 'NONE',  ( 3.458734125000001658, 4.235727675282972223E-16, 12.18750000136560629 ) ) ;
#8575=ORIENTED_EDGE ( 'NONE', *, *, #13667, .T. ) ;
#8598=CARTESIAN_POINT ( 'NONE',  ( -3.458734124999998105, 1.432654583217640276, 13.37500000136560274 ) ) ;
#8605=EDGE_CURVE ( 'NONE', #18572, #10729, #12554, .T. ) ;
#8607=CARTESIAN_POINT ( 'NONE',  ( 9.920644283265380691E-16, 4.000000000000000000, 13.87500000273119483 ) ) ;
#8618=CARTESIAN_POINT ( 'NONE',  ( -2.828427124746189403, 2.828427124746190291, 11.87500000000001066 ) ) ;
#8626=CARTESIAN_POINT ( 'NONE',  ( 3.458734125000002102, -1.432654583217639610, 10.87500000136560452 ) ) ;
#8637=CARTESIAN_POINT ( 'NONE',  ( -3.458734124999998993, 0.000000000000000000, 19.43750000136560629 ) ) ;
#8645=CARTESIAN_POINT ( 'NONE',  ( 1.432654583217643163, -3.458734124999999882, 11.00000000136560452 ) ) ;
#8661=CARTESIAN_POINT ( 'NONE',  ( 3.458734125000001214, 1.432654583217640498, 18.00000000136560274 ) ) ;
#8664=EDGE_CURVE ( 'NONE', #19956, #4420, #3643, .T. ) ;
#8667=VERTEX_POINT ( 'NONE', #18612 ) ;
#8682=CARTESIAN_POINT ( 'NONE',  ( -3.458734124999999437, 0.000000000000000000, 15.68750000136560629 ) ) ;
#8683=CARTESIAN_POINT ( 'NONE',  ( 9.920644283265380691E-16, 4.000000000000000000, 10.87500000273119660 ) ) ;
#8688=CARTESIAN_POINT ( 'NONE',  ( 9.920644283265380691E-16, 4.000000000000000000, 18.87500000273119838 ) ) ;
#8693=CARTESIAN_POINT ( 'NONE',  ( 1.025207404391860050E-15, 3.458734125000000770, 10.43750000136560629 ) ) ;
#8715=CARTESIAN_POINT ( 'NONE',  ( -3.458734124999998105, -1.432654583217642275, 15.50000000136560807 ) ) ;
#8745=CARTESIAN_POINT ( 'NONE',  ( 3.458734125000001658, 4.235727675282972223E-16, 18.18750000136560274 ) ) ;
#8751=CARTESIAN_POINT ( 'NONE',  ( -3.999999999999999112, 1.656854249492380582, 11.06250000273119660 ) ) ;
#8761=ADVANCED_FACE ( 'NONE', ( #21724 ), #14586, .T. ) ;
#8764=EDGE_CURVE ( 'NONE', #20917, #12579, #3884, .T. ) ;
#8766=CARTESIAN_POINT ( 'NONE',  ( -3.999999999999998224, -1.656854249492383246, 18.06250000000001421 ) ) ;
#8781=CARTESIAN_POINT ( 'NONE',  ( 9.920644283265380691E-16, 4.000000000000000000, 9.875000002731196602 ) ) ;
#8801=ORIENTED_EDGE ( 'NONE', *, *, #22768, .T. ) ;
#8805=VECTOR ( 'NONE', #13237, 1000.000000000000000 ) ;
#8810=CARTESIAN_POINT ( 'NONE',  ( 3.458734125000001658, 4.235727675282972223E-16, 14.18750000136560629 ) ) ;
#8811=CARTESIAN_POINT ( 'NONE',  ( -1.656854249492379250, 4.000000000000000000, 9.937500002731198379 ) ) ;
#8829=CARTESIAN_POINT ( 'NONE',  ( 4.000000000000000888, 4.898587196589412829E-16, 17.50000000000001066 ) ) ;
#8832=( BOUNDED_CURVE ( )  B_SPLINE_CURVE ( 2, ( #13708, #2538, #756, #4590, #20969, #11925, #3497, #15964, #23021 ),
 .UNSPECIFIED., .F., .F. ) 
 B_SPLINE_CURVE_WITH_KNOTS ( ( 3, 2, 2, 2, 3 ),
 ( 0.2000000000000000111, 0.2124999999999999944, 0.2250000000000000056, 0.2374999999999999889, 0.2500000000000000000 ),
 .UNSPECIFIED. ) 
 CURVE ( )  GEOMETRIC_REPRESENTATION_ITEM ( )  RATIONAL_B_SPLINE_CURVE ( ( 1.000000000000000000, 0.9238795325112867385, 1.000000000000000000, 0.9238795325112867385, 1.000000000000000000, 0.9238795325112867385, 1.000000000000000000, 0.9238795325112867385, 1.000000000000000000 ) ) 
 REPRESENTATION_ITEM ( '' )  );
#8837=CARTESIAN_POINT ( 'NONE',  ( -1.656854249492380138, -3.999999999999999112, 12.18750000000001066 ) ) ;
#8844=CARTESIAN_POINT ( 'NONE',  ( 1.656854249492384135, -3.999999999999999112, 17.43750000273119483 ) ) ;
#8848=CARTESIAN_POINT ( 'NONE',  ( -1.432654583217639610, -3.458734124999999882, 16.62500000136560629 ) ) ;
#8859=ORIENTED_EDGE ( 'NONE', *, *, #4571, .F. ) ;
#8876=CARTESIAN_POINT ( 'NONE',  ( 1.432654583217641386, 3.458734125000000770, 17.37500000136560274 ) ) ;
#8880=PLANE ( 'NONE',  #7413 ) ;
#8882=CARTESIAN_POINT ( 'NONE',  ( -3.999999999999999112, 0.000000000000000000, 11.12500000273119660 ) ) ;
#8891=CARTESIAN_POINT ( 'NONE',  ( -1.656854249492380138, -3.999999999999999112, 17.18750000000001066 ) ) ;
#8899=DIRECTION ( 'NONE',  ( -0.000000000000000000, 0.000000000000000000, -1.000000000000000000 ) ) ;
#8904=CARTESIAN_POINT ( 'NONE',  ( 3.458734125000001214, 1.432654583217640498, 19.00000000136560629 ) ) ;
#8908=CARTESIAN_POINT ( 'NONE',  ( 1.656854249492384135, -3.999999999999999112, 14.43750000273119660 ) ) ;
#8915=ORIENTED_EDGE ( 'NONE', *, *, #21597, .F. ) ;
#8926=CARTESIAN_POINT ( 'NONE',  ( -2.445694354108818303, -2.445694354108820967, 16.81250000136560629 ) ) ;
#8949=CARTESIAN_POINT ( 'NONE',  ( -3.999999999999999112, 0.000000000000000000, 17.00000000000001066 ) ) ;
#8955=CARTESIAN_POINT ( 'NONE',  ( -3.999999999999998224, -1.656854249492383246, 11.06250000000001066 ) ) ;
#8967=CARTESIAN_POINT ( 'NONE',  ( -3.458734124999998105, -1.432654583217642275, 13.50000000136560452 ) ) ;
#8975=CARTESIAN_POINT ( 'NONE',  ( 4.000000000000000888, 4.898587196589412829E-16, 21.31370849898476649 ) ) ;
#8980=CARTESIAN_POINT ( 'NONE',  ( 1.656854249492381470, 4.000000000000000000, 13.81250000273119483 ) ) ;
#8992=CARTESIAN_POINT ( 'NONE',  ( 1.656854249492381470, 4.000000000000000000, 15.81250000273119660 ) ) ;
#8995=LINE ( 'NONE', #18071, #3398 ) ;
#8997=LINE ( 'NONE', #5026, #16133 ) ;
#9012=CARTESIAN_POINT ( 'NONE',  ( -1.656854249492379250, 4.000000000000000000, 16.81250000000001066 ) ) ;
#9016=DIRECTION ( 'NONE',  ( 0.9413949561959079615, 0.3373062947069096484, -0.000000000000000000 ) ) ;
#9022=CARTESIAN_POINT ( 'NONE',  ( 3.458734125000001214, 4.235727675282971730E-16, 17.93750000136560274 ) ) ;
#9027=CARTESIAN_POINT ( 'NONE',  ( 1.432654583217641164, 3.458734125000000326, 16.12500000136560629 ) ) ;
#9045=CARTESIAN_POINT ( 'NONE',  ( -3.458734124999999437, 1.432654583217640498, 13.62500000136560452 ) ) ;
#9053=CARTESIAN_POINT ( 'NONE',  ( -0.3649867057748841237, 3.983313282257322285, 21.31370849898476649 ) ) ;
#9055=ORIENTED_EDGE ( 'NONE', *, *, #2676, .F. ) ;
#9061=CARTESIAN_POINT ( 'NONE',  ( -2.828427124746188515, -2.828427124746190735, 18.12500000000001066 ) ) ;
#9064=CARTESIAN_POINT ( 'NONE',  ( -2.247776618166720475, 3.308700692843488333, 9.970592379354943802 ) ) ;
#9091=CARTESIAN_POINT ( 'NONE',  ( 4.000000000000001776, -1.656854249492379694, 18.43750000000001066 ) ) ;
#9093=VECTOR ( 'NONE', #2077, 1000.000000000000000 ) ;
#9100=EDGE_CURVE ( 'NONE', #20911, #14597, #5869, .T. ) ;
#9102=CARTESIAN_POINT ( 'NONE',  ( -2.828427124746189403, 2.828427124746190291, 17.00000000273119838 ) ) ;
#9110=AXIS2_PLACEMENT_3D ( 'NONE', #15434, #21010, #15554 ) ;
#9129=CARTESIAN_POINT ( 'NONE',  ( -1.432654583217639166, 3.458734125000000770, 10.50000000136560629 ) ) ;
#9136=ADVANCED_FACE ( 'NONE', ( #16649 ), #1911, .F. ) ;
#9142=CARTESIAN_POINT ( 'NONE',  ( 1.432654583217641164, 3.458734125000000326, 18.12500000136560274 ) ) ;
#9147=CARTESIAN_POINT ( 'NONE',  ( 3.458734125000002102, -1.432654583217639610, 14.87500000136560807 ) ) ;
#9157=CARTESIAN_POINT ( 'NONE',  ( -1.656854249492380138, -3.999999999999999112, 17.18750000000001066 ) ) ;
#9163=VECTOR ( 'NONE', #11406, 1000.000000000000000 ) ;
#9168=CARTESIAN_POINT ( 'NONE',  ( 1.432654583217643163, -3.458734124999999882, 13.00000000136560629 ) ) ;
#9179=CYLINDRICAL_SURFACE ( 'NONE', #7177, 4.000000000000000000 ) ;
#9186=EDGE_CURVE ( 'NONE', #15974, #18318, #7197, .T. ) ;
#9187=CARTESIAN_POINT ( 'NONE',  ( -3.999999999999999112, 1.656854249492380804, 15.93750000000001066 ) ) ;
#9203=CARTESIAN_POINT ( 'NONE',  ( 4.000000000000001776, -1.656854249492379694, 18.56250000273119838 ) ) ;
#9205=CARTESIAN_POINT ( 'NONE',  ( -2.828427124746189403, 2.828427124746190291, 16.87500000000001066 ) ) ;
#9216=ORIENTED_EDGE ( 'NONE', *, *, #2676, .T. ) ;
#9223=CARTESIAN_POINT ( 'NONE',  ( -3.999999999999998224, -1.656854249492383024, 16.06250000000001066 ) ) ;
#9226=CARTESIAN_POINT ( 'NONE',  ( -3.999999999999999112, -2.265485919601331943, 19.21045885948849019 ) ) ;
#9246=EDGE_LOOP ( 'NONE', ( #20597, #7800, #13125, #15727 ) ) ;
#9249=CARTESIAN_POINT ( 'NONE',  ( 1.656854249492381470, 4.000000000000000000, 17.68750000000001066 ) ) ;
#9254=DIRECTION ( 'NONE',  ( -0.3373062947069096484, 0.9413949561959079615, 0.000000000000000000 ) ) ;
#9259=CARTESIAN_POINT ( 'NONE',  ( -3.458734124999998993, -1.432654583217642497, 16.50000000136560629 ) ) ;
#9264=CARTESIAN_POINT ( 'NONE',  ( -3.458734124999998993, 0.000000000000000000, 12.43750000136560629 ) ) ;
#9268=ORIENTED_EDGE ( 'NONE', *, *, #10738, .F. ) ;
#9276=CARTESIAN_POINT ( 'NONE',  ( 2.445694354108821411, 2.445694354108820523, 19.31250000136560629 ) ) ;
#9280=CARTESIAN_POINT ( 'NONE',  ( 3.458734125000001658, 1.432654583217640498, 12.25000000136560629 ) ) ;
#9285=CARTESIAN_POINT ( 'NONE',  ( 9.920644283265380691E-16, 4.000000000000000000, 17.87500000273119483 ) ) ;
#9295=EDGE_CURVE ( 'NONE', #7848, #20461, #2384, .T. ) ;
#9298=CARTESIAN_POINT ( 'NONE',  ( -1.656854249492379250, 4.000000000000000000, 18.81250000000001776 ) ) ;
#9310=CARTESIAN_POINT ( 'NONE',  ( -1.432654583217639166, 3.458734125000000770, 15.50000000136560807 ) ) ;
#9311=DIRECTION ( 'NONE',  ( 1.000000000000000000, 0.000000000000000000, -1.224646799147353207E-16 ) ) ;
#9317=VERTEX_POINT ( 'NONE', #20700 ) ;
#9324=ORIENTED_EDGE ( 'NONE', *, *, #20632, .T. ) ;
#9329=CARTESIAN_POINT ( 'NONE',  ( 4.000000000000000888, 1.656854249492381248, 19.56250000000001421 ) ) ;
#9334=CARTESIAN_POINT ( 'NONE',  ( -1.656854249492379250, 4.000000000000000000, 17.93750000273119483 ) ) ;
#9344=CARTESIAN_POINT ( 'NONE',  ( 4.000000000000000888, 4.898587196589412829E-16, 18.50000000000001066 ) ) ;
#9356=CARTESIAN_POINT ( 'NONE',  ( 1.656854249492381470, 4.000000000000000000, 15.68750000000001066 ) ) ;
#9361=CARTESIAN_POINT ( 'NONE',  ( 2.828427124746191179, 2.828427124746190291, 17.75000000273119483 ) ) ;
#9368=CARTESIAN_POINT ( 'NONE',  ( 3.458734125000002102, -1.432654583217639610, 15.87500000136560807 ) ) ;
#9370=AXIS2_PLACEMENT_3D ( 'NONE', #4375, #11713, #20881 ) ;
#9374=CARTESIAN_POINT ( 'NONE',  ( -2.445694354108819191, 2.445694354108820523, 13.31250000136560452 ) ) ;
#9383=ORIENTED_EDGE ( 'NONE', *, *, #22864, .T. ) ;
#9386=CARTESIAN_POINT ( 'NONE',  ( 3.458734125000002546, -1.432654583217639610, 16.12500000136560629 ) ) ;
#9388=AXIS2_PLACEMENT_3D ( 'NONE', #22842, #6454, #3165 ) ;
#9390=EDGE_CURVE ( 'NONE', #16438, #14597, #21399, .T. ) ;
#9392=CARTESIAN_POINT ( 'NONE',  ( -3.458734124999999437, 1.432654583217640498, 10.62500000136560807 ) ) ;
#9397=EDGE_CURVE ( 'NONE', #22113, #7929, #10077, .T. ) ;
#9399=CARTESIAN_POINT ( 'NONE',  ( -3.458734124999998993, 0.000000000000000000, 10.43750000136560452 ) ) ;
#9400=CARTESIAN_POINT ( 'NONE',  ( 2.828427124746192067, -2.828427124746189847, 16.50000000273119838 ) ) ;
#9412=CARTESIAN_POINT ( 'NONE',  ( 1.971781867644420635E-15, -4.000000000000000000, 13.25000000000001243 ) ) ;
#9427=CARTESIAN_POINT ( 'NONE',  ( -3.458734124999999437, 1.432654583217640498, 13.62500000136560452 ) ) ;
#9429=CARTESIAN_POINT ( 'NONE',  ( 1.656854249492381470, 4.000000000000000000, 16.68750000000001066 ) ) ;
#9431=CARTESIAN_POINT ( 'NONE',  ( 4.000000000000000888, 4.898587196589412829E-16, 17.50000000000001066 ) ) ;
#9444=( BOUNDED_CURVE ( )  B_SPLINE_CURVE ( 2, ( #23130, #10477, #3376, #8908, #19540, #14050, #8549, #17758, #5171 ),
 .UNSPECIFIED., .F., .F. ) 
 B_SPLINE_CURVE_WITH_KNOTS ( ( 3, 2, 2, 2, 3 ),
 ( 0.4500000000000000111, 0.4625000000000000222, 0.4749999999999999778, 0.4874999999999999889, 0.5000000000000000000 ),
 .UNSPECIFIED. ) 
 CURVE ( )  GEOMETRIC_REPRESENTATION_ITEM ( )  RATIONAL_B_SPLINE_CURVE ( ( 1.000000000000000000, 0.9238795325112867385, 1.000000000000000000, 0.9238795325112867385, 1.000000000000000000, 0.9238795325112867385, 1.000000000000000000, 0.9238795325112867385, 1.000000000000000000 ) ) 
 REPRESENTATION_ITEM ( '' )  );
#9447=CARTESIAN_POINT ( 'NONE',  ( -1.656854249492379250, 4.000000000000000000, 10.81250000000001243 ) ) ;
#9465=CARTESIAN_POINT ( 'NONE',  ( -3.999999999999998224, -1.656854249492383024, 16.18750000273119838 ) ) ;
#9467=FACE_OUTER_BOUND ( 'NONE', #15836, .T. ) ;
#9471=CARTESIAN_POINT ( 'NONE',  ( -2.828427124746188515, -2.828427124746190735, 13.12500000000001243 ) ) ;
#9481=CARTESIAN_POINT ( 'NONE',  ( -1.432654583217638944, 3.458734125000000326, 18.25000000136560629 ) ) ;
#9485=CARTESIAN_POINT ( 'NONE',  ( 9.920644283265380691E-16, 4.000000000000000000, 12.75000000000001066 ) ) ;
#9486=CARTESIAN_POINT ( 'NONE',  ( -1.432654583217638944, 3.458734125000000326, 13.25000000136560452 ) ) ;
#9495=SHAPE_DEFINITION_REPRESENTATION ( #17381, #20612 ) ;
#9503=CARTESIAN_POINT ( 'NONE',  ( -1.432654583217639166, 3.458734125000000770, 15.50000000136560807 ) ) ;
#9504=EDGE_CURVE ( 'NONE', #21075, #10762, #4958, .T. ) ;
#9511=CARTESIAN_POINT ( 'NONE',  ( -1.432654583217639832, -3.458734125000000326, 11.87500000136560629 ) ) ;
#9519=CARTESIAN_POINT ( 'NONE',  ( 1.872352939448454495E-15, -3.458734125000000326, 10.68750000136560452 ) ) ;
#9520=CARTESIAN_POINT ( 'NONE',  ( 1.656854249492381470, 4.000000000000000000, 14.81250000273119483 ) ) ;
#9524=EDGE_CURVE ( 'NONE', #4420, #13926, #5339, .T. ) ;
#9525=DIRECTION ( 'NONE',  ( -1.000000000000000000, 0.000000000000000000, 0.000000000000000000 ) ) ;
#9532=CARTESIAN_POINT ( 'NONE',  ( -3.999999999999999112, 1.656854249492380804, 11.93750000000001066 ) ) ;
#9537=EDGE_CURVE ( 'NONE', #7575, #1132, #7558, .T. ) ;
#9549=CARTESIAN_POINT ( 'NONE',  ( 3.458734125000001658, 4.235727675282972223E-16, 15.18750000136560452 ) ) ;
#9550=CARTESIAN_POINT ( 'NONE',  ( -20.00000000000001066, 9.999999999999964473, -49.99999999999999289 ) ) ;
#9553=DIRECTION ( 'NONE',  ( -0.000000000000000000, -0.000000000000000000, -1.000000000000000000 ) ) ;
#9554=ORIENTED_EDGE ( 'NONE', *, *, #19677, .T. ) ;
#9574=CARTESIAN_POINT ( 'NONE',  ( -3.999999999999999112, 0.000000000000000000, 20.00000000000001066 ) ) ;
#9578=CARTESIAN_POINT ( 'NONE',  ( 4.000000000000000888, 4.898587196589412829E-16, 13.62500000273119660 ) ) ;
#9583=VECTOR ( 'NONE', #15034, 1000.000000000000000 ) ;
#9602=PLANE ( 'NONE',  #11052 ) ;
#9604=CARTESIAN_POINT ( 'NONE',  ( -3.999999999999998224, -1.656854249492383246, 16.06250000000001066 ) ) ;
#9615=CARTESIAN_POINT ( 'NONE',  ( -2.445694354108818303, -2.445694354108820523, 12.56250000136560629 ) ) ;
#9620=CARTESIAN_POINT ( 'NONE',  ( -3.458734124999998993, 0.000000000000000000, 13.43750000136560452 ) ) ;
#9629=DIRECTION ( 'NONE',  ( 0.000000000000000000, 0.000000000000000000, -1.000000000000000000 ) ) ;
#9630=ORIENTED_EDGE ( 'NONE', *, *, #21834, .F. ) ;
#9633=CARTESIAN_POINT ( 'NONE',  ( 3.458734125000001658, 4.235727675282972223E-16, 15.18750000136560452 ) ) ;
#9643=CARTESIAN_POINT ( 'NONE',  ( 1.025207404391860050E-15, 3.458734125000000326, 10.18750000136560629 ) ) ;
#9644=CARTESIAN_POINT ( 'NONE',  ( -1.656854249492379250, 4.000000000000000000, 15.93750000273119838 ) ) ;
#9655=CARTESIAN_POINT ( 'NONE',  ( 1.971781867644420635E-15, -4.000000000000000000, 12.25000000000001066 ) ) ;
#9669=CARTESIAN_POINT ( 'NONE',  ( -3.458734124999998993, -1.432654583217642497, 14.75000000136560452 ) ) ;
#9679=FACE_OUTER_BOUND ( 'NONE', #8526, .T. ) ;
#9689=CARTESIAN_POINT ( 'NONE',  ( -1.656854249492380138, -3.999999999999999112, 12.31250000273119660 ) ) ;
#9694=CARTESIAN_POINT ( 'NONE',  ( -3.458734124999998105, 1.432654583217640276, 17.37500000136560274 ) ) ;
#9699=ORIENTED_EDGE ( 'NONE', *, *, #15085, .T. ) ;
#9702=ORIENTED_EDGE ( 'NONE', *, *, #3203, .T. ) ;
#9703=VECTOR ( 'NONE', #5737, 1000.000000000000000 ) ;
#9706=CARTESIAN_POINT ( 'NONE',  ( -3.999999999999999112, 0.000000000000000000, 11.12500000273119660 ) ) ;
#9711=CARTESIAN_POINT ( 'NONE',  ( 4.000000000000000888, 4.898587196589412829E-16, 18.62500000273119483 ) ) ;
#9712=CARTESIAN_POINT ( 'NONE',  ( -1.656854249492379250, 4.000000000000000000, 15.81250000000001066 ) ) ;
#9720=DIRECTION ( 'NONE',  ( 0.000000000000000000, 0.000000000000000000, 1.000000000000000000 ) ) ;
#9723=CARTESIAN_POINT ( 'NONE',  ( 1.872352939448454495E-15, -3.458734125000000326, 13.68750000136560629 ) ) ;
#9732=ORIENTED_EDGE ( 'NONE', *, *, #636, .T. ) ;
#9737=PRODUCT_CONTEXT ( 'NONE', #14678, 'mechanical' ) ;
#9743=CARTESIAN_POINT ( 'NONE',  ( -2.445694354108819191, 2.445694354108820523, 16.56250000136560629 ) ) ;
#9752=CARTESIAN_POINT ( 'NONE',  ( -1.432654583217639610, -3.458734124999999882, 10.62500000136560452 ) ) ;
#9753=CARTESIAN_POINT ( 'NONE',  ( 4.000000000000000888, 1.656854249492381248, 13.68750000273119483 ) ) ;
#9756=CYLINDRICAL_SURFACE ( 'NONE', #10527, 4.999999999999997335 ) ;
#9764=CARTESIAN_POINT ( 'NONE',  ( -2.828427124746189403, 2.828427124746190291, 12.87500000000001066 ) ) ;
#9768=VERTEX_POINT ( 'NONE', #18773 ) ;
#9774=B_SPLINE_CURVE_WITH_KNOTS ( 'NONE', 1,
 ( #5918, #16471 ),
 .UNSPECIFIED., .F., .F.,
 ( 2, 2 ),
 ( 0.000000000000000000, 1.000000000000000000 ),
 .UNSPECIFIED. ) ;
#9782=CARTESIAN_POINT ( 'NONE',  ( 1.872352939448454495E-15, -3.458734125000000770, 13.93750000136560629 ) ) ;
#9791=ORIENTED_EDGE ( 'NONE', *, *, #20632, .F. ) ;
#9794=EDGE_CURVE ( 'NONE', #12677, #3140, #13405, .T. ) ;
#9796=EDGE_LOOP ( 'NONE', ( #19107, #13340, #1196, #10839 ) ) ;
#9809=CARTESIAN_POINT ( 'NONE',  ( 1.432654583217641164, 3.458734125000000326, 19.12500000136560629 ) ) ;
#9829=CARTESIAN_POINT ( 'NONE',  ( -3.999999999999999112, 0.000000000000000000, 15.00000000000001066 ) ) ;
#9832=ADVANCED_FACE ( 'NONE', ( #4154 ), #16307, .T. ) ;
#9838=CARTESIAN_POINT ( 'NONE',  ( -2.828427124746188515, -2.828427124746190735, 10.25000000273119660 ) ) ;
#9840=CARTESIAN_POINT ( 'NONE',  ( -2.445694354108818303, -2.445694354108820523, 13.56250000136560629 ) ) ;
#9860=CARTESIAN_POINT ( 'NONE',  ( 1.432654583217641386, 3.458734125000000770, 18.37500000136560274 ) ) ;
#9875=CARTESIAN_POINT ( 'NONE',  ( 1.872352939448454495E-15, -3.458734125000000326, 12.68750000136560629 ) ) ;
#9876=CARTESIAN_POINT ( 'NONE',  ( 1.971781867644420635E-15, -4.000000000000000000, 11.37500000273119660 ) ) ;
#9878=PLANE ( 'NONE',  #16469 ) ;
#9880=VECTOR ( 'NONE', #13274, 1000.000000000000000 ) ;
#9888=ORIENTED_EDGE ( 'NONE', *, *, #12319, .T. ) ;
#9889=CARTESIAN_POINT ( 'NONE',  ( -2.828427124746189403, 2.828427124746190291, 14.87500000000000888 ) ) ;
#9899=DIRECTION ( 'NONE',  ( -0.000000000000000000, -0.000000000000000000, -1.000000000000000000 ) ) ;
#9901=CARTESIAN_POINT ( 'NONE',  ( 1.025207404391860050E-15, 3.458734125000000770, 18.43750000136560629 ) ) ;
#9902=CARTESIAN_POINT ( 'NONE',  ( 1.656854249492384135, -3.999999999999999112, 11.31250000000001066 ) ) ;
#9907=CARTESIAN_POINT ( 'NONE',  ( -2.445694354108819191, 2.445694354108820523, 11.56250000136560629 ) ) ;
#9917=ORIENTED_EDGE ( 'NONE', *, *, #110, .F. ) ;
#9930=DIRECTION ( 'NONE',  ( -0.000000000000000000, -0.000000000000000000, -1.000000000000000000 ) ) ;
#9934=CARTESIAN_POINT ( 'NONE',  ( 1.025207404391860050E-15, 3.458734125000000326, 18.18750000136560274 ) ) ;
#9945=CIRCLE ( 'NONE', #3791, 4.000000000000000000 ) ;
#9955=CARTESIAN_POINT ( 'NONE',  ( -3.999999999999998224, -1.656854249492383246, 12.06250000000001243 ) ) ;
#9966=CARTESIAN_POINT ( 'NONE',  ( -3.999999999999999112, 0.000000000000000000, 21.31370849898476649 ) ) ;
#9968=CARTESIAN_POINT ( 'NONE',  ( 1.025207404391860050E-15, 3.458734125000000326, 12.18750000136560629 ) ) ;
#9974=CARTESIAN_POINT ( 'NONE',  ( -3.999999999999999112, 1.656854249492380582, 15.93750000000001066 ) ) ;
#9976=CARTESIAN_POINT ( 'NONE',  ( -2.762848947613219419, 4.746226468750993632, -19.99999999999999645 ) ) ;
#9977=EDGE_CURVE ( 'NONE', #5706, #6890, #5542, .T. ) ;
#9979=ORIENTED_EDGE ( 'NONE', *, *, #8208, .F. ) ;
#9989=CARTESIAN_POINT ( 'NONE',  ( -3.458734124999999437, 1.432654583217640498, 13.62500000136560452 ) ) ;
#9993=VECTOR ( 'NONE', #19385, 1000.000000000000114 ) ;
#10003=CARTESIAN_POINT ( 'NONE',  ( -2.828427124746188515, -2.828427124746190735, 10.25000000273119660 ) ) ;
#10009=CARTESIAN_POINT ( 'NONE',  ( 4.000000000000000888, 4.898587196589412829E-16, 13.50000000000001066 ) ) ;
#10025=CARTESIAN_POINT ( 'NONE',  ( 1.656854249492384135, -3.999999999999999112, 15.31250000000001243 ) ) ;
#10027=CARTESIAN_POINT ( 'NONE',  ( -2.445694354108818303, -2.445694354108820967, 17.81250000136560274 ) ) ;
#10039=CARTESIAN_POINT ( 'NONE',  ( -35.00000000000000000, 7.500000000000001776, -19.99999999999998934 ) ) ;
#10049=PRODUCT_DEFINITION_CONTEXT ( 'detailed design', #3943, 'design' ) ;
#10056=CARTESIAN_POINT ( 'NONE',  ( -3.458734124999998993, 0.000000000000000000, 19.43750000136560629 ) ) ;
#10059=ORIENTED_EDGE ( 'NONE', *, *, #12888, .T. ) ;
#10060=LINE ( 'NONE', #17350, #383 ) ;
#10077=LINE ( 'NONE', #6584, #1114 ) ;
#10082=DIRECTION ( 'NONE',  ( 0.000000000000000000, -1.000000000000000000, 0.000000000000000000 ) ) ;
#10084=CARTESIAN_POINT ( 'NONE',  ( 2.445694354108821411, 2.445694354108820523, 14.06250000136560452 ) ) ;
#10090=CARTESIAN_POINT ( 'NONE',  ( -1.432654583217639610, -3.458734124999999882, 10.62500000136560274 ) ) ;
#10092=VERTEX_POINT ( 'NONE', #22172 ) ;
#10103=CARTESIAN_POINT ( 'NONE',  ( -3.458734124999998993, -1.432654583217642497, 12.75000000136560629 ) ) ;
#10115=CARTESIAN_POINT ( 'NONE',  ( -1.656854249492380138, -3.999999999999999112, 13.31250000273119660 ) ) ;
#10138=CARTESIAN_POINT ( 'NONE',  ( 1.236993788156008760E-15, 0.000000000000000000, 21.31370849898476649 ) ) ;
#10139=CARTESIAN_POINT ( 'NONE',  ( -3.458734124999999437, 0.000000000000000000, 19.68750000136560629 ) ) ;
#10140=CARTESIAN_POINT ( 'NONE',  ( 1.656854249492381470, 4.000000000000000000, 11.81250000273119838 ) ) ;
#10153=CARTESIAN_POINT ( 'NONE',  ( 1.971781867644420635E-15, -4.000000000000000000, 14.25000000000001066 ) ) ;
#10154=AXIS2_PLACEMENT_3D ( 'NONE', #22873, #2401, #953 ) ;
#10155=SURFACE_SIDE_STYLE ('',( #1242 ) ) ;
#10163=DIRECTION ( 'NONE',  ( -1.224646799147353207E-16, 0.000000000000000000, -1.000000000000000000 ) ) ;
#10176=CARTESIAN_POINT ( 'NONE',  ( -2.445694354108819191, 2.445694354108820523, 17.31250000136560274 ) ) ;
#10179=EDGE_LOOP ( 'NONE', ( #20572, #9554, #5897, #5862 ) ) ;
#10180=FACE_BOUND ( 'NONE', #18775, .T. ) ;
#10200=VECTOR ( 'NONE', #19394, 1000.000000000000000 ) ;
#10202=CARTESIAN_POINT ( 'NONE',  ( -3.999999999999999112, 0.000000000000000000, 10.12500000273119660 ) ) ;
#10204=CARTESIAN_POINT ( 'NONE',  ( -1.432654583217639832, -3.458734125000000326, 18.87500000136560274 ) ) ;
#10221=CARTESIAN_POINT ( 'NONE',  ( -3.458734124999999437, 0.000000000000000000, 13.68750000136560629 ) ) ;
#10234=CARTESIAN_POINT ( 'NONE',  ( -14.99999999999996980, 15.00000000000000000, -19.99999999999999645 ) ) ;
#10235=CARTESIAN_POINT ( 'NONE',  ( 9.920644283265380691E-16, 4.000000000000000000, 12.87500000273119660 ) ) ;
#10239=CARTESIAN_POINT ( 'NONE',  ( -3.999999999999999112, 1.656854249492380582, 13.93750000000001243 ) ) ;
#10248=CARTESIAN_POINT ( 'NONE',  ( 4.000000000000000888, 1.656854249492381248, 19.56250000000001421 ) ) ;
#10255=CARTESIAN_POINT ( 'NONE',  ( 3.458734125000001658, 4.235727675282972223E-16, 18.18750000136560274 ) ) ;
#10256=CARTESIAN_POINT ( 'NONE',  ( -2.828427124746189403, 2.828427124746190291, 15.00000000273119660 ) ) ;
#10280=FACE_OUTER_BOUND ( 'NONE', #12954, .T. ) ;
#10295=CARTESIAN_POINT ( 'NONE',  ( 3.458734125000001214, 1.432654583217640498, 13.00000000136560452 ) ) ;
#10297=VECTOR ( 'NONE', #3022, 1000.000000000000000 ) ;
#10307=CARTESIAN_POINT ( 'NONE',  ( -3.999999999999999112, 1.656854249492380582, 14.06250000273119660 ) ) ;
#10314=CARTESIAN_POINT ( 'NONE',  ( -2.828427124746189403, 2.828427124746190291, 17.87500000000001066 ) ) ;
#10317=AXIS2_PLACEMENT_3D ( 'NONE', #17120, #15109, #15348 ) ;
#10325=CARTESIAN_POINT ( 'NONE',  ( 1.025207404391860050E-15, 3.458734125000000326, 11.18750000136560452 ) ) ;
#10331=CARTESIAN_POINT ( 'NONE',  ( 4.000000000000000888, 1.656854249492381248, 15.56250000000001066 ) ) ;
#10346=CARTESIAN_POINT ( 'NONE',  ( 2.445694354108821411, 2.445694354108820523, 11.31250000136560452 ) ) ;
#10358=CARTESIAN_POINT ( 'NONE',  ( -2.445694354108819191, 2.445694354108820523, 18.31250000136560274 ) ) ;
#10374=VERTEX_POINT ( 'NONE', #19644 ) ;
#10381=CARTESIAN_POINT ( 'NONE',  ( -3.458734124999998105, -1.432654583217642497, 15.75000000136560629 ) ) ;
#10382=CARTESIAN_POINT ( 'NONE',  ( -3.999999999999999112, 1.656854249492380804, 13.06250000273119660 ) ) ;
#10391=CARTESIAN_POINT ( 'NONE',  ( 1.872352939448454495E-15, -3.458734125000000770, 12.93750000136560629 ) ) ;
#10414=( BOUNDED_CURVE ( )  B_SPLINE_CURVE ( 2, ( #11521, #15695, #19249, #15344, #18901, #8146, #11867, #4175, #9706 ),
 .UNSPECIFIED., .F., .F. ) 
 B_SPLINE_CURVE_WITH_KNOTS ( ( 3, 2, 2, 2, 3 ),
 ( 0.7500000000000000000, 0.7624999999999999556, 0.7750000000000000222, 0.7874999999999999778, 0.8000000000000000444 ),
 .UNSPECIFIED. ) 
 CURVE ( )  GEOMETRIC_REPRESENTATION_ITEM ( )  RATIONAL_B_SPLINE_CURVE ( ( 1.000000000000000000, 0.9238795325112867385, 1.000000000000000000, 0.9238795325112867385, 1.000000000000000000, 0.9238795325112867385, 1.000000000000000000, 0.9238795325112867385, 1.000000000000000000 ) ) 
 REPRESENTATION_ITEM ( '' )  );
#10418=CARTESIAN_POINT ( 'NONE',  ( 1.025207404391860050E-15, 3.458734125000000326, 15.18750000136560452 ) ) ;
#10436=CARTESIAN_POINT ( 'NONE',  ( -3.999999999999999112, 0.000000000000000000, 19.00000000000001066 ) ) ;
#10437=CARTESIAN_POINT ( 'NONE',  ( -3.999999999999999112, 1.656854249492380582, 11.93750000000001066 ) ) ;
#10445=CARTESIAN_POINT ( 'NONE',  ( -2.445694354108819191, 2.445694354108820523, 11.31250000136560452 ) ) ;
#10461=CARTESIAN_POINT ( 'NONE',  ( 3.458734125000001658, 1.432654583217640498, 13.25000000136560452 ) ) ;
#10470=LINE ( 'NONE', #10823, #18485 ) ;
#10472=CARTESIAN_POINT ( 'NONE',  ( 1.971781867644420635E-15, -4.000000000000000000, 13.25000000000001243 ) ) ;
#10473=CARTESIAN_POINT ( 'NONE',  ( 19.99999999999998934, -9.999999999999964473, -50.00000000000000000 ) ) ;
#10474=CARTESIAN_POINT ( 'NONE',  ( 1.432654583217643163, -3.458734124999999437, 15.75000000136560629 ) ) ;
#10477=CARTESIAN_POINT ( 'NONE',  ( 4.000000000000001776, -1.656854249492379694, 14.56250000273119660 ) ) ;
#10478=VERTEX_POINT ( 'NONE', #20466 ) ;
#10482=CARTESIAN_POINT ( 'NONE',  ( 27.50000000000000000, 4.500000000000001776, -33.66025403784446723 ) ) ;
#10494=CARTESIAN_POINT ( 'NONE',  ( 2.445694354108821411, 2.445694354108820523, 17.31250000136560629 ) ) ;
#10495=CARTESIAN_POINT ( 'NONE',  ( 2.828427124746191179, 2.828427124746190291, 10.75000000273119660 ) ) ;
#10527=AXIS2_PLACEMENT_3D ( 'NONE', #13835, #20855, #21090 ) ;
#10531=CARTESIAN_POINT ( 'NONE',  ( 2.445694354108821411, 2.445694354108820523, 15.06250000136560452 ) ) ;
#10548=VECTOR ( 'NONE', #23673, 1000.000000000000000 ) ;
#10561=CARTESIAN_POINT ( 'NONE',  ( 2.445694354108822299, -2.445694354108820079, 18.06250000136560274 ) ) ;
#10568=EDGE_CURVE ( 'NONE', #10092, #12579, #4071, .T. ) ;
#10578=ORIENTED_EDGE ( 'NONE', *, *, #5962, .T. ) ;
#10580=ADVANCED_FACE ( 'NONE', ( #18560 ), #3594, .T. ) ;
#10581=CARTESIAN_POINT ( 'NONE',  ( 2.828427124746191179, 2.828427124746190291, 12.75000000273119660 ) ) ;
#10583=CARTESIAN_POINT ( 'NONE',  ( 9.920644283265380691E-16, 4.000000000000000000, 17.75000000000000711 ) ) ;
#10596=LINE ( 'NONE', #16199, #5757 ) ;
#10597=CARTESIAN_POINT ( 'NONE',  ( -3.458734124999998993, 1.432654583217640276, 18.37500000136560274 ) ) ;
#10600=DIRECTION ( 'NONE',  ( -0.3373062947069096484, 0.9413949561959079615, 0.000000000000000000 ) ) ;
#10607=VERTEX_POINT ( 'NONE', #2273 ) ;
#10617=CARTESIAN_POINT ( 'NONE',  ( -3.458734124999998105, -1.432654583217642497, 14.75000000136560452 ) ) ;
#10646=LINE ( 'NONE', #5103, #14553 ) ;
#10650=CARTESIAN_POINT ( 'NONE',  ( 3.458734125000001214, 4.235727675282971730E-16, 15.93750000136560629 ) ) ;
#10668=EDGE_CURVE ( 'NONE', #22004, #4764, #18328, .T. ) ;
#10679=CARTESIAN_POINT ( 'NONE',  ( 1.025207404391860050E-15, 3.458734125000000770, 17.43750000136560274 ) ) ;
#10685=CARTESIAN_POINT ( 'NONE',  ( 2.828427124746191179, 2.828427124746190291, 10.75000000273119660 ) ) ;
#10686=DIRECTION ( 'NONE',  ( 0.000000000000000000, 0.000000000000000000, 1.000000000000000000 ) ) ;
#10691=CARTESIAN_POINT ( 'NONE',  ( -3.999999999999999112, 0.000000000000000000, 21.31370849898476649 ) ) ;
#10692=EDGE_LOOP ( 'NONE', ( #7939, #7682, #18034, #13360 ) ) ;
#10695=CARTESIAN_POINT ( 'NONE',  ( 2.828427124746191179, 2.828427124746190291, 19.62500000000001066 ) ) ;
#10697=EDGE_CURVE ( 'NONE', #17674, #7114, #17351, .T. ) ;
#10708=EDGE_CURVE ( 'NONE', #7114, #1597, #17134, .T. ) ;
#10713=CARTESIAN_POINT ( 'NONE',  ( 1.872352939448454495E-15, -3.458734125000000326, 16.68750000136560629 ) ) ;
#10729=VERTEX_POINT ( 'NONE', #6114 ) ;
#10736=CARTESIAN_POINT ( 'NONE',  ( 1.025207404391860050E-15, 3.458734125000000770, 16.43750000136560629 ) ) ;
#10737=CARTESIAN_POINT ( 'NONE',  ( 2.828427124746192067, -2.828427124746189847, 11.50000000273119660 ) ) ;
#10738=EDGE_CURVE ( 'NONE', #15974, #18572, #4548, .T. ) ;
#10746=CARTESIAN_POINT ( 'NONE',  ( 4.000000000000000888, 4.898587196589412829E-16, 18.62500000273119483 ) ) ;
#10748=AXIS2_PLACEMENT_3D ( 'NONE', #15210, #6570, #13528 ) ;
#10756=CARTESIAN_POINT ( 'NONE',  ( 1.656854249492384135, -3.999999999999999112, 18.31250000000001421 ) ) ;
#10761=CARTESIAN_POINT ( 'NONE',  ( 1.971781867644420635E-15, -4.000000000000000000, 12.25000000000001066 ) ) ;
#10762=VERTEX_POINT ( 'NONE', #22742 ) ;
#10768=ADVANCED_FACE ( 'NONE', ( #15361, #22628 ), #6231, .F. ) ;
#10773=CARTESIAN_POINT ( 'NONE',  ( -2.445694354108818303, -2.445694354108820523, 14.56250000136560452 ) ) ;
#10774=CARTESIAN_POINT ( 'NONE',  ( -1.656854249492380138, -3.999999999999999112, 18.31250000273119483 ) ) ;
#10779=CARTESIAN_POINT ( 'NONE',  ( -0.3649867057748643617, 3.983313282257324950, 10.00000000000000888 ) ) ;
#10785=CARTESIAN_POINT ( 'NONE',  ( -3.999999999999999112, 0.000000000000000000, 16.12500000273119838 ) ) ;
#10793=CARTESIAN_POINT ( 'NONE',  ( 4.000000000000000888, 1.656854249492381248, 16.68750000273119838 ) ) ;
#10815=CARTESIAN_POINT ( 'NONE',  ( -3.999999999999999112, 0.000000000000000000, 13.12500000273119660 ) ) ;
#10816=CARTESIAN_POINT ( 'NONE',  ( -3.999999999999999112, 0.000000000000000000, 17.00000000000001066 ) ) ;
#10819=CARTESIAN_POINT ( 'NONE',  ( 4.000000000000000888, 4.898587196589412829E-16, 21.31370849898476649 ) ) ;
#10820=DIRECTION ( 'NONE',  ( -0.000000000000000000, -0.000000000000000000, -1.000000000000000000 ) ) ;
#10823=CARTESIAN_POINT ( 'NONE',  ( -3.999999999999999112, 0.000000000000000000, 21.31370849898476649 ) ) ;
#10828=CARTESIAN_POINT ( 'NONE',  ( -3.458734124999998993, 1.432654583217640276, 16.37500000136560629 ) ) ;
#10831=EDGE_CURVE ( 'NONE', #4495, #6890, #3212, .T. ) ;
#10839=ORIENTED_EDGE ( 'NONE', *, *, #16016, .F. ) ;
#10840=EDGE_LOOP ( 'NONE', ( #5622, #12483 ) ) ;
#10841=FACE_OUTER_BOUND ( 'NONE', #795, .T. ) ;
#10846=CARTESIAN_POINT ( 'NONE',  ( -3.458734124999999437, 0.000000000000000000, 13.68750000136560629 ) ) ;
#10849=CARTESIAN_POINT ( 'NONE',  ( -27.50000000000000711, 7.500000000000001776, -33.66025403784446723 ) ) ;
#10851=CARTESIAN_POINT ( 'NONE',  ( 4.000000000000000888, 4.898587196589412829E-16, 15.62500000273119660 ) ) ;
#10860=EDGE_CURVE ( 'NONE', #3586, #1384, #8995, .T. ) ;
#10863=CARTESIAN_POINT ( 'NONE',  ( 2.828427124746191179, 2.828427124746190291, 17.62500000000001066 ) ) ;
#10880=CARTESIAN_POINT ( 'NONE',  ( 1.872352939448454495E-15, -3.458734125000000326, 11.68750000136560629 ) ) ;
#10903=CARTESIAN_POINT ( 'NONE',  ( 4.000000000000000888, 4.898587196589412829E-16, 17.62500000273119483 ) ) ;
#10911=CARTESIAN_POINT ( 'NONE',  ( -20.00000000000001066, 9.999999999999964473, -49.99999999999999289 ) ) ;
#10915=ORIENTED_EDGE ( 'NONE', *, *, #17141, .F. ) ;
#10920=EDGE_CURVE ( 'NONE', #7848, #3586, #16048, .T. ) ;
#10923=CYLINDRICAL_SURFACE ( 'NONE', #22106, 4.000000000000000000 ) ;
#10925=DIRECTION ( 'NONE',  ( -1.000000000000000000, 0.000000000000000000, 0.000000000000000000 ) ) ;
#10926=CARTESIAN_POINT ( 'NONE',  ( 1.872352939448454495E-15, -3.458734125000000770, 10.93750000136560452 ) ) ;
#10935=CARTESIAN_POINT ( 'NONE',  ( 3.458734125000001214, 4.235727675282971730E-16, 18.93750000136560629 ) ) ;
#10938=CARTESIAN_POINT ( 'NONE',  ( -1.970342311631612331, 3.497176594775547542, 10.00018359407915192 ) ) ;
#10939=CARTESIAN_POINT ( 'NONE',  ( 3.458734125000001214, 4.235727675282971730E-16, 13.93750000136560629 ) ) ;
#10940=CARTESIAN_POINT ( 'NONE',  ( 27.50000000000000000, 7.500000000000002665, -33.66025403784446723 ) ) ;
#10941=ORIENTED_EDGE ( 'NONE', *, *, #2258, .F. ) ;
#10958=CARTESIAN_POINT ( 'NONE',  ( 1.025207404391860050E-15, 3.458734125000000770, 10.43750000136560629 ) ) ;
#10959=CARTESIAN_POINT ( 'NONE',  ( -3.999999999999999112, 0.000000000000000000, 10.12500000273119660 ) ) ;
#10961=CARTESIAN_POINT ( 'NONE',  ( -0.1828748004095307189, 4.000000000000000000, 9.881898421846274871 ) ) ;
#10971=SHAPE_REPRESENTATION_RELATIONSHIP ( 'NONE' , 'NONE' ,  #20612, #19027 ) ;
#10975=CARTESIAN_POINT ( 'NONE',  ( -2.828427124746188515, -2.828427124746190735, 16.12500000000001066 ) ) ;
#10979=DIRECTION ( 'NONE',  ( 0.000000000000000000, -0.000000000000000000, -1.000000000000000000 ) ) ;
#10985=CARTESIAN_POINT ( 'NONE',  ( 19.99999999999998934, 7.500000000000002665, -50.00000000000000000 ) ) ;
#10993=CARTESIAN_POINT ( 'NONE',  ( -3.999999999999999112, 0.000000000000000000, 21.31370849898476649 ) ) ;
#10994=ORIENTED_EDGE ( 'NONE', *, *, #7239, .T. ) ;
#10997=CARTESIAN_POINT ( 'NONE',  ( -0.3649867057748917842, 3.983313282257320509, 9.889028792932920808 ) ) ;
#11014=CARTESIAN_POINT ( 'NONE',  ( 4.000000000000001776, -1.656854249492379694, 18.56250000273119838 ) ) ;
#11039=CARTESIAN_POINT ( 'NONE',  ( -3.999999999999998224, -1.656854249492383246, 19.06250000000001421 ) ) ;
#11044=ORIENTED_EDGE ( 'NONE', *, *, #19315, .F. ) ;
#11050=CARTESIAN_POINT ( 'NONE',  ( 2.445694354108821855, -2.445694354108820079, 18.81250000136560629 ) ) ;
#11052=AXIS2_PLACEMENT_3D ( 'NONE', #4417, #19366, #2961 ) ;
#11055=CARTESIAN_POINT ( 'NONE',  ( -3.458734124999998993, 1.432654583217640276, 15.37500000136560807 ) ) ;
#11064=AXIS2_PLACEMENT_3D ( 'NONE', #7681, #22249, #1781 ) ;
#11074=CARTESIAN_POINT ( 'NONE',  ( -3.458734124999999437, 0.000000000000000000, 10.68750000136560452 ) ) ;
#11080=CARTESIAN_POINT ( 'NONE',  ( -1.656854249492380138, -3.999999999999999112, 17.31250000273119483 ) ) ;
#11082=LINE ( 'NONE', #16936, #8805 ) ;
#11093=CARTESIAN_POINT ( 'NONE',  ( 4.000000000000001776, -1.656854249492379694, 17.43750000000001421 ) ) ;
#11112=CARTESIAN_POINT ( 'NONE',  ( -3.458734124999999437, 1.432654583217640498, 14.62500000136560629 ) ) ;
#11120=ORIENTED_EDGE ( 'NONE', *, *, #19407, .F. ) ;
#11123=EDGE_CURVE ( 'NONE', #12919, #12610, #11255, .T. ) ;
#11137=( BOUNDED_CURVE ( )  B_SPLINE_CURVE ( 2, ( #725, #21065, #491, #7814, #17028, #2516, #11420, #15132, #6004 ),
 .UNSPECIFIED., .F., .F. ) 
 B_SPLINE_CURVE_WITH_KNOTS ( ( 3, 2, 2, 2, 3 ),
 ( 0.2999999999999999889, 0.3125000000000000000, 0.3250000000000000111, 0.3375000000000000222, 0.3499999999999999778 ),
 .UNSPECIFIED. ) 
 CURVE ( )  GEOMETRIC_REPRESENTATION_ITEM ( )  RATIONAL_B_SPLINE_CURVE ( ( 1.000000000000000000, 0.9238795325112867385, 1.000000000000000000, 0.9238795325112867385, 1.000000000000000000, 0.9238795325112867385, 1.000000000000000000, 0.9238795325112867385, 1.000000000000000000 ) ) 
 REPRESENTATION_ITEM ( '' )  );
#11140=CARTESIAN_POINT ( 'NONE',  ( -3.999999999999999112, 0.000000000000000000, 16.12500000273119838 ) ) ;
#11148=ORIENTED_EDGE ( 'NONE', *, *, #14362, .T. ) ;
#11149=DIRECTION ( 'NONE',  ( -0.000000000000000000, -0.000000000000000000, -1.000000000000000000 ) ) ;
#11154=ORIENTED_EDGE ( 'NONE', *, *, #10860, .T. ) ;
#11160=ORIENTED_EDGE ( 'NONE', *, *, #22661, .T. ) ;
#11161=DIRECTION ( 'NONE',  ( -0.000000000000000000, -0.000000000000000000, -1.000000000000000000 ) ) ;
#11164=CARTESIAN_POINT ( 'NONE',  ( 4.000000000000000888, 4.898587196589412829E-16, 16.50000000000001066 ) ) ;
#11165=ADVANCED_FACE ( 'NONE', ( #15094 ), #22349, .T. ) ;
#11166=DIRECTION ( 'NONE',  ( -0.000000000000000000, -0.000000000000000000, -1.000000000000000000 ) ) ;
#11168=EDGE_CURVE ( 'NONE', #12677, #14904, #8190, .T. ) ;
#11170=CARTESIAN_POINT ( 'NONE',  ( -1.656854249492379472, 4.000000000000000000, 17.93750000273119483 ) ) ;
#11171=PLANE ( 'NONE',  #11438 ) ;
#11176=CARTESIAN_POINT ( 'NONE',  ( -2.445694354108819191, 2.445694354108820523, 17.31250000136560274 ) ) ;
#11181=CARTESIAN_POINT ( 'NONE',  ( 3.458734125000001214, 4.235727675282971730E-16, 11.93750000136560629 ) ) ;
#11191=ORIENTED_EDGE ( 'NONE', *, *, #8764, .F. ) ;
#11198=CARTESIAN_POINT ( 'NONE',  ( -2.445694354108818303, -2.445694354108820967, 10.81250000136560452 ) ) ;
#11203=CARTESIAN_POINT ( 'NONE',  ( -3.999999999999999112, 0.000000000000000000, 14.12500000273119660 ) ) ;
#11214=CARTESIAN_POINT ( 'NONE',  ( 1.656854249492381470, 4.000000000000000000, 17.68750000000001066 ) ) ;
#11227=CARTESIAN_POINT ( 'NONE',  ( 1.025207404391860050E-15, 3.458734125000000770, 15.43750000136560452 ) ) ;
#11246=DIRECTION ( 'NONE',  ( -0.000000000000000000, -0.000000000000000000, -1.000000000000000000 ) ) ;
#11250=CARTESIAN_POINT ( 'NONE',  ( -2.828427124746188515, -2.828427124746190735, 11.12500000000001066 ) ) ;
#11255=LINE ( 'NONE', #5374, #14984 ) ;
#11269=CARTESIAN_POINT ( 'NONE',  ( 2.828427124746192067, -2.828427124746189847, 16.50000000273119838 ) ) ;
#11275=CARTESIAN_POINT ( 'NONE',  ( 4.000000000000001776, -1.656854249492379694, 16.43750000000001066 ) ) ;
#11288=CARTESIAN_POINT ( 'NONE',  ( 2.445694354108821855, -2.445694354108820079, 16.81250000136560629 ) ) ;
#11294=CARTESIAN_POINT ( 'NONE',  ( 1.432654583217641164, 3.458734125000000326, 15.12500000136560807 ) ) ;
#11306=VERTEX_POINT ( 'NONE', #12534 ) ;
#11308=CARTESIAN_POINT ( 'NONE',  ( 1.872352939448454495E-15, -3.458734125000000770, 18.93750000136560629 ) ) ;
#11316=CARTESIAN_POINT ( 'NONE',  ( -3.458734124999999437, 1.432654583217640498, 12.62500000136560629 ) ) ;
#11324=CARTESIAN_POINT ( 'NONE',  ( 3.458734125000001214, 1.432654583217640498, 12.00000000136560807 ) ) ;
#11325=CARTESIAN_POINT ( 'NONE',  ( 2.828427124746192067, -2.828427124746189847, 15.50000000273119660 ) ) ;
#11338=CARTESIAN_POINT ( 'NONE',  ( -3.999999999999999112, 0.000000000000000000, 15.00000000000001066 ) ) ;
#11340=DIRECTION ( 'NONE',  ( -0.000000000000000000, -0.000000000000000000, -1.000000000000000000 ) ) ;
#11351=CARTESIAN_POINT ( 'NONE',  ( -1.432654583217639832, -3.458734125000000326, 13.87500000136560452 ) ) ;
#11368=CARTESIAN_POINT ( 'NONE',  ( 9.920644283265380691E-16, 4.000000000000000000, 19.75000000000001066 ) ) ;
#11371=CARTESIAN_POINT ( 'NONE',  ( -3.999999999999999112, 0.000000000000000000, 14.12500000273119660 ) ) ;
#11388=CARTESIAN_POINT ( 'NONE',  ( 4.000000000000000888, 4.898587196589412829E-16, 11.50000000000001066 ) ) ;
#11396=CARTESIAN_POINT ( 'NONE',  ( 1.971781867644420635E-15, -4.000000000000000000, 13.25000000000001243 ) ) ;
#11402=ADVANCED_FACE ( 'NONE', ( #15597 ), #832, .T. ) ;
#11406=DIRECTION ( 'NONE',  ( 1.224646799147353207E-16, 0.000000000000000000, 1.000000000000000000 ) ) ;
#11409=CARTESIAN_POINT ( 'NONE',  ( 3.458734125000001214, 4.235727675282971730E-16, 16.93750000136560629 ) ) ;
#11416=CARTESIAN_POINT ( 'NONE',  ( 2.445694354108821855, -2.445694354108820079, 12.81250000136560629 ) ) ;
#11417=DIRECTION ( 'NONE',  ( -1.000000000000000000, 0.000000000000000000, 0.000000000000000000 ) ) ;
#11420=CARTESIAN_POINT ( 'NONE',  ( 2.828427124746191179, 2.828427124746190291, 15.75000000273119660 ) ) ;
#11430=EDGE_CURVE ( 'NONE', #7815, #19956, #4315, .T. ) ;
#11433=CARTESIAN_POINT ( 'NONE',  ( -3.458734124999998993, -1.432654583217642497, 18.75000000136560274 ) ) ;
#11438=AXIS2_PLACEMENT_3D ( 'NONE', #23364, #9016, #9254 ) ;
#11446=CARTESIAN_POINT ( 'NONE',  ( -3.458734124999998105, 1.432654583217640276, 11.37500000136560452 ) ) ;
#11447=CARTESIAN_POINT ( 'NONE',  ( 1.656854249492384135, -3.999999999999999112, 14.43750000273119483 ) ) ;
#11457=CARTESIAN_POINT ( 'NONE',  ( -1.656854249492380138, -3.999999999999999112, 14.18750000000001066 ) ) ;
#11470=VECTOR ( 'NONE', #3839, 1000.000000000000000 ) ;
#11476=CARTESIAN_POINT ( 'NONE',  ( -1.432654583217639832, -3.458734125000000326, 15.87500000136560807 ) ) ;
#11480=CARTESIAN_POINT ( 'NONE',  ( 4.000000000000000888, 1.656854249492381248, 16.56250000000001066 ) ) ;
#11483=COLOUR_RGB ( '', 0.09019608, 0.27058824, 0.51372549) ;
#11494=ORIENTED_EDGE ( 'NONE', *, *, #19315, .T. ) ;
#11501=CARTESIAN_POINT ( 'NONE',  ( 2.828427124746191179, 2.828427124746190291, 19.62500000000001066 ) ) ;
#11504=ORIENTED_EDGE ( 'NONE', *, *, #15603, .F. ) ;
#11505=CARTESIAN_POINT ( 'NONE',  ( 4.000000000000000888, 4.898587196589412829E-16, 12.62500000273119660 ) ) ;
#11515=CARTESIAN_POINT ( 'NONE',  ( 4.000000000000000888, 4.898587196589412829E-16, 12.50000000000001066 ) ) ;
#11521=CARTESIAN_POINT ( 'NONE',  ( 4.000000000000000888, 4.898587196589412829E-16, 11.62500000273119660 ) ) ;
#11528=CARTESIAN_POINT ( 'NONE',  ( -3.999999999999999112, 0.000000000000000000, 16.00000000000001066 ) ) ;
#11538=CARTESIAN_POINT ( 'NONE',  ( 1.432654583217643163, -3.458734124999999437, 14.75000000136560452 ) ) ;
#11551=ORIENTED_EDGE ( 'NONE', *, *, #9977, .T. ) ;
#11553=VERTEX_POINT ( 'NONE', #4553 ) ;
#11556=CARTESIAN_POINT ( 'NONE',  ( -1.432654583217639832, -3.458734125000000326, 15.87500000136560807 ) ) ;
#11568=CARTESIAN_POINT ( 'NONE',  ( 1.432654583217641164, 3.458734125000000326, 11.12500000136560452 ) ) ;
#11569=CARTESIAN_POINT ( 'NONE',  ( -3.999999999999999112, 1.656854249492380804, 14.06250000273119660 ) ) ;
#11579=CARTESIAN_POINT ( 'NONE',  ( -3.999999999999999112, 0.000000000000000000, 14.00000000000001066 ) ) ;
#11587=CARTESIAN_POINT ( 'NONE',  ( 3.458734125000001658, 4.235727675282972223E-16, 19.18750000136560629 ) ) ;
#11594=CARTESIAN_POINT ( 'NONE',  ( -3.458734124999999437, 0.000000000000000000, 15.68750000136560629 ) ) ;
#11603=EDGE_CURVE ( 'NONE', #19299, #19630, #7066, .T. ) ;
#11606=ORIENTED_EDGE ( 'NONE', *, *, #9295, .T. ) ;
#11611=CARTESIAN_POINT ( 'NONE',  ( 1.656854249492384135, -3.999999999999999112, 19.31250000000001776 ) ) ;
#11615=CARTESIAN_POINT ( 'NONE',  ( -20.00000000000000711, 7.500000000000002665, -19.99999999999999645 ) ) ;
#11632=CARTESIAN_POINT ( 'NONE',  ( 4.000000000000000888, 4.898587196589412829E-16, 14.62500000273119660 ) ) ;
#11640=CARTESIAN_POINT ( 'NONE',  ( -2.828427124746189403, 2.828427124746190291, 14.87500000000000888 ) ) ;
#11651=CARTESIAN_POINT ( 'NONE',  ( -2.445694354108819191, 2.445694354108820523, 14.31250000136560452 ) ) ;
#11657=CARTESIAN_POINT ( 'NONE',  ( 3.458734125000001214, 4.235727675282971730E-16, 10.93750000136560452 ) ) ;
#11660=PRODUCT ( 'motor', 'motor', '', ( #9737 ) ) ;
#11670=CARTESIAN_POINT ( 'NONE',  ( -3.458734124999999437, 0.000000000000000000, 18.68750000136560629 ) ) ;
#11681=CARTESIAN_POINT ( 'NONE',  ( 2.828427124746192067, -2.828427124746189847, 11.50000000273119660 ) ) ;
#11684=CARTESIAN_POINT ( 'NONE',  ( 1.656854249492381470, 4.000000000000000000, 13.68750000000001066 ) ) ;
#11691=CARTESIAN_POINT ( 'NONE',  ( 1.656854249492384135, -3.999999999999999112, 13.31250000000001243 ) ) ;
#11699=( BOUNDED_CURVE ( )  B_SPLINE_CURVE ( 2, ( #1053, #10437, #8618, #2616, #12109, #23086, #19371, #2965, #14012 ),
 .UNSPECIFIED., .F., .F. ) 
 B_SPLINE_CURVE_WITH_KNOTS ( ( 3, 2, 2, 2, 3 ),
 ( 0.8000000000000000444, 0.8125000000000000000, 0.8249999999999999556, 0.8375000000000000222, 0.8499999999999999778 ),
 .UNSPECIFIED. ) 
 CURVE ( )  GEOMETRIC_REPRESENTATION_ITEM ( )  RATIONAL_B_SPLINE_CURVE ( ( 1.000000000000000000, 0.9238795325112867385, 1.000000000000000000, 0.9238795325112867385, 1.000000000000000000, 0.9238795325112867385, 1.000000000000000000, 0.9238795325112867385, 1.000000000000000000 ) ) 
 REPRESENTATION_ITEM ( '' )  );
#11700=CARTESIAN_POINT ( 'NONE',  ( 1.872352939448454495E-15, -3.458734125000000770, 17.93750000136560274 ) ) ;
#11704=VECTOR ( 'NONE', #14449, 1000.000000000000000 ) ;
#11709=CARTESIAN_POINT ( 'NONE',  ( 3.458734125000001658, 1.432654583217640498, 11.25000000136560452 ) ) ;
#11713=DIRECTION ( 'NONE',  ( -1.224646799147353207E-16, 0.000000000000000000, -1.000000000000000000 ) ) ;
#11727=EDGE_CURVE ( 'NONE', #17599, #12610, #8997, .T. ) ;
#11728=AXIS2_PLACEMENT_3D ( 'NONE', #23313, #21379, #1511 ) ;
#11737=CARTESIAN_POINT ( 'NONE',  ( 1.432654583217643163, -3.458734124999999437, 18.75000000136560985 ) ) ;
#11748=ADVANCED_FACE ( 'NONE', ( #3921 ), #12939, .F. ) ;
#11763=CARTESIAN_POINT ( 'NONE',  ( 19.99999999999998934, 4.500000000000001776, -50.00000000000000000 ) ) ;
#11766=CARTESIAN_POINT ( 'NONE',  ( 1.025207404391860050E-15, 3.458734125000000326, 14.18750000136560452 ) ) ;
#11769=ORIENTED_EDGE ( 'NONE', *, *, #12888, .F. ) ;
#11784=CARTESIAN_POINT ( 'NONE',  ( 2.445694354108821411, 2.445694354108820523, 17.31250000136560629 ) ) ;
#11799=CARTESIAN_POINT ( 'NONE',  ( -1.656854249492380138, -3.999999999999999112, 12.31250000273119660 ) ) ;
#11805=ORIENTED_EDGE ( 'NONE', *, *, #5067, .F. ) ;
#11812=CARTESIAN_POINT ( 'NONE',  ( 4.000000000000000888, 1.656854249492381248, 14.56250000000000888 ) ) ;
#11814=AXIS2_PLACEMENT_3D ( 'NONE', #6942, #1527, #23570 ) ;
#11819=CARTESIAN_POINT ( 'NONE',  ( -1.432654583217639166, 3.458734125000000770, 19.50000000136560629 ) ) ;
#11832=CARTESIAN_POINT ( 'NONE',  ( 35.00000000000000000, 7.500000000000001776, -20.00000000000000355 ) ) ;
#11840=LINE ( 'NONE', #662, #9880 ) ;
#11841=ORIENTED_EDGE ( 'NONE', *, *, #19459, .T. ) ;
#11852=CARTESIAN_POINT ( 'NONE',  ( 4.000000000000000888, 4.898587196589412829E-16, 12.62500000273119660 ) ) ;
#11853=CARTESIAN_POINT ( 'NONE',  ( 3.458734125000001214, 4.235727675282971730E-16, 17.93750000136560274 ) ) ;
#11860=CARTESIAN_POINT ( 'NONE',  ( -2.828427124746188515, -2.828427124746190735, 12.12500000000001066 ) ) ;
#11867=CARTESIAN_POINT ( 'NONE',  ( -2.828427124746188515, -2.828427124746190735, 11.25000000273119660 ) ) ;
#11876=CARTESIAN_POINT ( 'NONE',  ( 1.656854249492384135, -3.999999999999999112, 12.31250000000001243 ) ) ;
#11883=DIRECTION ( 'NONE',  ( -1.000000000000000000, 0.000000000000000000, 0.000000000000000000 ) ) ;
#11886=CARTESIAN_POINT ( 'NONE',  ( -3.458734124999998993, -1.432654583217642497, 11.50000000136560629 ) ) ;
#11895=CARTESIAN_POINT ( 'NONE',  ( -1.432654583217638944, 3.458734125000000326, 11.25000000136560452 ) ) ;
#11907=CARTESIAN_POINT ( 'NONE',  ( -2.445694354108819191, 2.445694354108820523, 13.56250000136560629 ) ) ;
#11913=CARTESIAN_POINT ( 'NONE',  ( 35.00000000000000000, 4.500000000000001776, -20.00000000000000355 ) ) ;
#11921=CARTESIAN_POINT ( 'NONE',  ( -3.999999999999999112, 1.656854249492380804, 10.06250000273119660 ) ) ;
#11925=CARTESIAN_POINT ( 'NONE',  ( 1.656854249492381470, 4.000000000000000000, 16.81250000273119838 ) ) ;
#11931=ADVANCED_FACE ( 'NONE', ( #2365, #10180 ), #18894, .F. ) ;
#11937=ORIENTED_EDGE ( 'NONE', *, *, #9794, .T. ) ;
#11943=CARTESIAN_POINT ( 'NONE',  ( 4.000000000000000888, 4.898587196589412829E-16, 15.50000000000001066 ) ) ;
#11945=CARTESIAN_POINT ( 'NONE',  ( 4.000000000000001776, -1.656854249492379694, 12.56250000273119660 ) ) ;
#11951=CARTESIAN_POINT ( 'NONE',  ( -2.445694354108818303, -2.445694354108820967, 12.81250000136560629 ) ) ;
#11957=FILL_AREA_STYLE_COLOUR ( '', #13390 ) ;
#11991=CARTESIAN_POINT ( 'NONE',  ( -1.656854249492380138, -3.999999999999999112, 16.18750000000001066 ) ) ;
#11992=EDGE_CURVE ( 'NONE', #17728, #4019, #6449, .T. ) ;
#12000=CARTESIAN_POINT ( 'NONE',  ( -3.458734124999998993, 0.000000000000000000, 12.43750000136560629 ) ) ;
#12002=DIRECTION ( 'NONE',  ( 1.224646799147353207E-16, -0.000000000000000000, 1.000000000000000000 ) ) ;
#12017=CARTESIAN_POINT ( 'NONE',  ( 3.458734125000002546, -1.432654583217639610, 13.12500000136560629 ) ) ;
#12019=VECTOR ( 'NONE', #5080, 1000.000000000000000 ) ;
#12024=DIRECTION ( 'NONE',  ( -0.000000000000000000, -0.000000000000000000, -1.000000000000000000 ) ) ;
#12034=CARTESIAN_POINT ( 'NONE',  ( 1.656854249492381470, 4.000000000000000000, 12.81250000273119660 ) ) ;
#12042=FACE_OUTER_BOUND ( 'NONE', #14930, .T. ) ;
#12044=CARTESIAN_POINT ( 'NONE',  ( -0.9413949561959078505, -0.3373062947069096484, 10.00000000000000888 ) ) ;
#12049=( BOUNDED_CURVE ( )  B_SPLINE_CURVE ( 2, ( #23123, #17523, #14045, #4933, #10472, #12142, #6850, #21197, #4811 ),
 .UNSPECIFIED., .F., .F. ) 
 B_SPLINE_CURVE_WITH_KNOTS ( ( 3, 2, 2, 2, 3 ),
 ( 0.6500000000000000222, 0.6624999999999999778, 0.6750000000000000444, 0.6875000000000000000, 0.6999999999999999556 ),
 .UNSPECIFIED. ) 
 CURVE ( )  GEOMETRIC_REPRESENTATION_ITEM ( )  RATIONAL_B_SPLINE_CURVE ( ( 1.000000000000000000, 0.9238795325112867385, 1.000000000000000000, 0.9238795325112867385, 1.000000000000000000, 0.9238795325112867385, 1.000000000000000000, 0.9238795325112867385, 1.000000000000000000 ) ) 
 REPRESENTATION_ITEM ( '' )  );
#12050=EDGE_CURVE ( 'NONE', #12476, #21889, #10060, .T. ) ;
#12053=CARTESIAN_POINT ( 'NONE',  ( 1.025207404391860050E-15, 3.458734125000000770, 19.43750000136560629 ) ) ;
#12054=CARTESIAN_POINT ( 'NONE',  ( 1.656854249492384135, -3.999999999999999112, 14.43750000273119483 ) ) ;
#12061=CARTESIAN_POINT ( 'NONE',  ( -3.458734124999998993, -1.432654583217642497, 11.75000000136560629 ) ) ;
#12083=ORIENTED_EDGE ( 'NONE', *, *, #21051, .T. ) ;
#12088=CARTESIAN_POINT ( 'NONE',  ( -2.445694354108818303, -2.445694354108820523, 13.56250000136560629 ) ) ;
#12104=CARTESIAN_POINT ( 'NONE',  ( 19.99999999999999289, 9.999999999999966249, -20.00000000000000355 ) ) ;
#12109=CARTESIAN_POINT ( 'NONE',  ( 9.920644283265380691E-16, 4.000000000000000000, 11.75000000000001066 ) ) ;
#12112=CARTESIAN_POINT ( 'NONE',  ( -15.00000000000000711, -10.00000000000000000, -19.99999999999999645 ) ) ;
#12115=CARTESIAN_POINT ( 'NONE',  ( -2.445694354108818303, -2.445694354108820523, 10.56250000136560452 ) ) ;
#12126=EDGE_LOOP ( 'NONE', ( #17418, #3440, #6132, #11551 ) ) ;
#12129=LINE ( 'NONE', #12489, #10200 ) ;
#12132=CARTESIAN_POINT ( 'NONE',  ( -1.432654583217639166, 3.458734125000000770, 11.50000000136560629 ) ) ;
#12142=CARTESIAN_POINT ( 'NONE',  ( -1.656854249492380138, -3.999999999999999112, 13.18750000000001243 ) ) ;
#12144=CARTESIAN_POINT ( 'NONE',  ( 2.828427124746192067, -2.828427124746189847, 13.50000000273119660 ) ) ;
#12165=CARTESIAN_POINT ( 'NONE',  ( 2.445694354108822299, -2.445694354108820079, 17.06250000136560629 ) ) ;
#12166=CARTESIAN_POINT ( 'NONE',  ( 2.828427124746191179, 2.828427124746190291, 12.75000000273119660 ) ) ;
#12188=VECTOR ( 'NONE', #1281, 1000.000000000000000 ) ;
#12201=CARTESIAN_POINT ( 'NONE',  ( 1.971781867644420635E-15, -4.000000000000000000, 17.37500000273119483 ) ) ;
#12205=CARTESIAN_POINT ( 'NONE',  ( -3.458734124999998105, -1.432654583217642275, 16.50000000136560629 ) ) ;
#12208=CARTESIAN_POINT ( 'NONE',  ( -3.999999999999999112, 0.000000000000000000, 12.00000000000001066 ) ) ;
#12209=EDGE_LOOP ( 'NONE', ( #4424, #11191, #12466, #13836 ) ) ;
#12232=VERTEX_POINT ( 'NONE', #9431 ) ;
#12238=CARTESIAN_POINT ( 'NONE',  ( -2.445694354108819191, 2.445694354108820523, 18.56250000136560629 ) ) ;
#12245=CARTESIAN_POINT ( 'NONE',  ( 27.50000000000000000, 4.500000000000001776, -33.66025403784446723 ) ) ;
#12250=ORIENTED_EDGE ( 'NONE', *, *, #2597, .T. ) ;
#12255=CARTESIAN_POINT ( 'NONE',  ( 3.458734125000002546, -1.432654583217639610, 12.12500000136560629 ) ) ;
#12270=CARTESIAN_POINT ( 'NONE',  ( -1.432654583217638944, 3.458734125000000326, 18.25000000136560629 ) ) ;
#12274=DIRECTION ( 'NONE',  ( 0.000000000000000000, -0.000000000000000000, 1.000000000000000000 ) ) ;
#12282=CARTESIAN_POINT ( 'NONE',  ( 14.99999999999995559, 15.00000000000000000, -50.00000000000000000 ) ) ;
#12292=CARTESIAN_POINT ( 'NONE',  ( -3.458734124999998105, -1.432654583217642497, 16.75000000136560629 ) ) ;
#12303=EDGE_LOOP ( 'NONE', ( #18139, #50, #4028, #7290 ) ) ;
#12311=DIRECTION ( 'NONE',  ( 0.000000000000000000, 0.000000000000000000, 1.000000000000000000 ) ) ;
#12314=AXIS2_PLACEMENT_3D ( 'NONE', #5965, #6325, #13763 ) ;
#12315=CARTESIAN_POINT ( 'NONE',  ( 2.828427124746192067, -2.828427124746189847, 12.37500000000001066 ) ) ;
#12319=EDGE_CURVE ( 'NONE', #14904, #10478, #2646, .T. ) ;
#12327=CARTESIAN_POINT ( 'NONE',  ( 3.458734125000002102, -1.432654583217639610, 14.87500000136560807 ) ) ;
#12329=EDGE_CURVE ( 'NONE', #14633, #2992, #14569, .T. ) ;
#12335=CARTESIAN_POINT ( 'NONE',  ( 1.236993788156008760E-15, 0.000000000000000000, -20.00000000000000000 ) ) ;
#12354=CARTESIAN_POINT ( 'NONE',  ( 1.025207404391860050E-15, 3.458734125000000770, 18.43750000136560629 ) ) ;
#12372=CARTESIAN_POINT ( 'NONE',  ( -1.432654583217639166, 3.458734125000000770, 14.50000000136560629 ) ) ;
#12384=CARTESIAN_POINT ( 'NONE',  ( 2.445694354108821855, -2.445694354108820079, 17.81250000136560274 ) ) ;
#12385=CARTESIAN_POINT ( 'NONE',  ( -3.729367062499998831, 0.000000000000000000, 19.84375000068280670 ) ) ;
#12387=PLANE ( 'NONE',  #13577 ) ;
#12398=CARTESIAN_POINT ( 'NONE',  ( 34.99999999999999289, 7.500000000000001776, -50.00000000000000000 ) ) ;
#12402=CARTESIAN_POINT ( 'NONE',  ( -0.8800590352214046064, 5.420839058164813373, -26.84672628368516811 ) ) ;
#12404=CARTESIAN_POINT ( 'NONE',  ( -3.458734124999999437, 0.000000000000000000, 14.68750000136560452 ) ) ;
#12407=CYLINDRICAL_SURFACE ( 'NONE', #20149, 2.649999999999992806 ) ;
#12413=LINE ( 'NONE', #19679, #5625 ) ;
#12428=SURFACE_STYLE_FILL_AREA ( #14097 ) ;
#12439=CARTESIAN_POINT ( 'NONE',  ( -1.432654583217639610, -3.458734124999999882, 15.62500000136560629 ) ) ;
#12440=CARTESIAN_POINT ( 'NONE',  ( 1.971781867644420635E-15, -4.000000000000000000, 18.37500000273119483 ) ) ;
#12450=EDGE_CURVE ( 'NONE', #10374, #13219, #13104, .T. ) ;
#12455=ORIENTED_EDGE ( 'NONE', *, *, #20930, .F. ) ;
#12466=ORIENTED_EDGE ( 'NONE', *, *, #12662, .F. ) ;
#12472=CARTESIAN_POINT ( 'NONE',  ( -3.458734124999999437, 0.000000000000000000, 17.68750000136560274 ) ) ;
#12476=VERTEX_POINT ( 'NONE', #15429 ) ;
#12483=ORIENTED_EDGE ( 'NONE', *, *, #20495, .F. ) ;
#12489=CARTESIAN_POINT ( 'NONE',  ( 19.99999999999999289, 9.999999999999964473, -20.00000000000000355 ) ) ;
#12494=CARTESIAN_POINT ( 'NONE',  ( 4.000000000000001776, -1.656854249492379694, 19.43750000000001066 ) ) ;
#12509=CARTESIAN_POINT ( 'NONE',  ( 3.458734125000001214, 4.235727675282971730E-16, 17.93750000136560274 ) ) ;
#12523=EDGE_CURVE ( 'NONE', #2255, #14480, #17216, .T. ) ;
#12529=CARTESIAN_POINT ( 'NONE',  ( -2.445694354108818303, -2.445694354108820967, 13.81250000136560629 ) ) ;
#12530=CARTESIAN_POINT ( 'NONE',  ( 4.000000000000000888, 4.898587196589412829E-16, 11.62500000273119660 ) ) ;
#12534=CARTESIAN_POINT ( 'NONE',  ( -3.999999999999999112, 0.000000000000000000, 19.12500000273119838 ) ) ;
#12535=CARTESIAN_POINT ( 'NONE',  ( -1.656854249492380138, -3.999999999999999112, 18.31250000273119838 ) ) ;
#12547=CARTESIAN_POINT ( 'NONE',  ( -2.828427124746189403, 2.828427124746190291, 17.87500000000001066 ) ) ;
#12554=LINE ( 'NONE', #3419, #7943 ) ;
#12560=CARTESIAN_POINT ( 'NONE',  ( 4.000000000000001776, -1.656854249492379694, 17.56250000273119483 ) ) ;
#12566=CARTESIAN_POINT ( 'NONE',  ( 1.432654583217641164, 3.458734125000000326, 16.12500000136560629 ) ) ;
#12579=VERTEX_POINT ( 'NONE', #17905 ) ;
#12580=CARTESIAN_POINT ( 'NONE',  ( -27.50000000000000711, 4.500000000000001776, -33.66025403784446723 ) ) ;
#12589=CARTESIAN_POINT ( 'NONE',  ( 2.828427124746192067, -2.828427124746189847, 17.50000000273119483 ) ) ;
#12609=DIRECTION ( 'NONE',  ( -0.3373062947069096484, 0.9413949561959079615, 0.000000000000000000 ) ) ;
#12610=VERTEX_POINT ( 'NONE', #8181 ) ;
#12611=CARTESIAN_POINT ( 'NONE',  ( -35.00000000000000000, 4.500000000000001776, -19.99999999999998934 ) ) ;
#12615=CARTESIAN_POINT ( 'NONE',  ( 4.000000000000000888, 4.898587196589412829E-16, 17.50000000000001066 ) ) ;
#12626=CARTESIAN_POINT ( 'NONE',  ( -3.458734124999999437, 0.000000000000000000, 19.68750000136560629 ) ) ;
#12632=CARTESIAN_POINT ( 'NONE',  ( -3.458734124999998993, 0.000000000000000000, 16.43750000136560629 ) ) ;
#12650=CARTESIAN_POINT ( 'NONE',  ( -2.445694354108818303, -2.445694354108820967, 14.81250000136560452 ) ) ;
#12651=CARTESIAN_POINT ( 'NONE',  ( 4.000000000000001776, -1.656854249492379694, 11.56250000273119838 ) ) ;
#12658=CARTESIAN_POINT ( 'NONE',  ( -2.828427124746189403, 2.828427124746190291, 18.00000000273119483 ) ) ;
#12662=EDGE_CURVE ( 'NONE', #18572, #20917, #13929, .T. ) ;
#12673=CARTESIAN_POINT ( 'NONE',  ( -3.999999999999998224, -1.656854249492383246, 18.06250000000001421 ) ) ;
#12677=VERTEX_POINT ( 'NONE', #17281 ) ;
#12678=PLANE ( 'NONE',  #12993 ) ;
#12679=DIRECTION ( 'NONE',  ( -1.000000000000000000, 0.000000000000000000, 0.000000000000000000 ) ) ;
#12680=EDGE_LOOP ( 'NONE', ( #14128, #17409, #4815, #13624 ) ) ;
#12685=CYLINDRICAL_SURFACE ( 'NONE', #20783, 4.000000000000000000 ) ;
#12690=CARTESIAN_POINT ( 'NONE',  ( -3.458734124999998105, 1.432654583217640276, 12.37500000136560629 ) ) ;
#12692=CARTESIAN_POINT ( 'NONE',  ( -3.999999999999998224, -1.656854249492383024, 18.18750000273119483 ) ) ;
#12699=EDGE_LOOP ( 'NONE', ( #6422, #2250, #5645, #23022 ) ) ;
#12713=CARTESIAN_POINT ( 'NONE',  ( 1.971781867644420635E-15, -4.000000000000000000, 17.37500000273119483 ) ) ;
#12725=ORIENTED_EDGE ( 'NONE', *, *, #455, .F. ) ;
#12729=ORIENTED_EDGE ( 'NONE', *, *, #8393, .T. ) ;
#12730=CARTESIAN_POINT ( 'NONE',  ( 1.236993788156008760E-15, 0.000000000000000000, 21.31370849898476649 ) ) ;
#12733=CARTESIAN_POINT ( 'NONE',  ( 4.000000000000000888, 4.898587196589412829E-16, 18.50000000000001066 ) ) ;
#12734=CARTESIAN_POINT ( 'NONE',  ( -2.828427124746189403, 2.828427124746190291, 18.87500000000001066 ) ) ;
#12742=CARTESIAN_POINT ( 'NONE',  ( -2.445694354108818303, -2.445694354108820523, 18.56250000136560629 ) ) ;
#12746=CARTESIAN_POINT ( 'NONE',  ( 1.025207404391860050E-15, 3.458734125000000326, 19.18750000136560629 ) ) ;
#12756=EDGE_CURVE ( 'NONE', #14629, #9317, #14164, .T. ) ;
#12764=CARTESIAN_POINT ( 'NONE',  ( -3.458734124999999437, 0.000000000000000000, 12.68750000136560629 ) ) ;
#12765=CARTESIAN_POINT ( 'NONE',  ( 2.828427124746192067, -2.828427124746189847, 10.50000000273119660 ) ) ;
#12781=CARTESIAN_POINT ( 'NONE',  ( 1.971781867644420635E-15, -4.000000000000000000, 18.25000000000001066 ) ) ;
#12808=ORIENTED_EDGE ( 'NONE', *, *, #5722, .T. ) ;
#12819=CARTESIAN_POINT ( 'NONE',  ( 2.828427124746192067, -2.828427124746189847, 18.50000000273119483 ) ) ;
#12833=CARTESIAN_POINT ( 'NONE',  ( 35.00000000000000000, 7.500000000000001776, -20.00000000000000355 ) ) ;
#12837=LINE ( 'NONE', #18434, #4931 ) ;
#12840=CARTESIAN_POINT ( 'NONE',  ( 2.828427124746191179, 2.828427124746190291, 16.62500000000001066 ) ) ;
#12841=DIRECTION ( 'NONE',  ( -0.000000000000000000, 1.000000000000000000, -0.000000000000000000 ) ) ;
#12842=CARTESIAN_POINT ( 'NONE',  ( -27.50000000000000711, 7.500000000000001776, -33.66025403784446723 ) ) ;
#12849=CARTESIAN_POINT ( 'NONE',  ( 2.445694354108821855, -2.445694354108820079, 17.81250000136560274 ) ) ;
#12854=CARTESIAN_POINT ( 'NONE',  ( 2.445694354108821411, 2.445694354108820523, 14.06250000136560452 ) ) ;
#12864=LINE ( 'NONE', #7463, #8260 ) ;
#12873=CARTESIAN_POINT ( 'NONE',  ( 1.872352939448454495E-15, -3.458734125000000770, 11.93750000136560629 ) ) ;
#12880=CARTESIAN_POINT ( 'NONE',  ( 4.000000000000001776, -1.656854249492379694, 15.56250000273119660 ) ) ;
#12882=EDGE_LOOP ( 'NONE', ( #189, #20832, #18369, #11120, #19828 ) ) ;
#12885=ORIENTED_EDGE ( 'NONE', *, *, #455, .T. ) ;
#12888=EDGE_CURVE ( 'NONE', #13665, #4526, #3589, .T. ) ;
#12891=CARTESIAN_POINT ( 'NONE',  ( 1.656854249492381470, 4.000000000000000000, 18.68750000000001066 ) ) ;
#12894=ORIENTED_EDGE ( 'NONE', *, *, #7773, .T. ) ;
#12896=CARTESIAN_POINT ( 'NONE',  ( 1.236993788156008760E-15, 0.000000000000000000, 21.31370849898476649 ) ) ;
#12899=EDGE_CURVE ( 'NONE', #11306, #10762, #20100, .T. ) ;
#12905=CARTESIAN_POINT ( 'NONE',  ( -3.458734124999999437, 1.432654583217640498, 16.62500000136560629 ) ) ;
#12919=VERTEX_POINT ( 'NONE', #2016 ) ;
#12923=VECTOR ( 'NONE', #21847, 1000.000000000000000 ) ;
#12930=CARTESIAN_POINT ( 'NONE',  ( -1.656854249492380138, -3.999999999999999112, 16.31250000273119483 ) ) ;
#12939=PLANE ( 'NONE',  #6945 ) ;
#12954=EDGE_LOOP ( 'NONE', ( #19274, #17787, #5713, #18344, #4563, #17188, #3352, #11148, #9216, #13408, #2517, #23075, #3406, #3906, #724, #8801 ) ) ;
#12957=CARTESIAN_POINT ( 'NONE',  ( 2.828427124746192067, -2.828427124746189847, 14.37500000000001066 ) ) ;
#12969=CARTESIAN_POINT ( 'NONE',  ( 3.458734125000001214, 1.432654583217640498, 18.00000000136560274 ) ) ;
#12974=CARTESIAN_POINT ( 'NONE',  ( -3.458734124999998993, -1.432654583217642497, 13.50000000136560452 ) ) ;
#12984=DIRECTION ( 'NONE',  ( -0.000000000000000000, -0.000000000000000000, -1.000000000000000000 ) ) ;
#12987=CARTESIAN_POINT ( 'NONE',  ( 1.432654583217643163, -3.458734124999999882, 19.00000000136560629 ) ) ;
#12993=AXIS2_PLACEMENT_3D ( 'NONE', #7269, #14585, #10979 ) ;
#12994=CARTESIAN_POINT ( 'NONE',  ( -3.458734124999999437, 0.000000000000000000, 11.68750000136560629 ) ) ;
#12998=CARTESIAN_POINT ( 'NONE',  ( -3.999999999999999112, 0.000000000000000000, 15.12500000273119660 ) ) ;
#13012=CARTESIAN_POINT ( 'NONE',  ( 4.000000000000000888, 4.898587196589412829E-16, 18.50000000000001066 ) ) ;
#13013=( GEOMETRIC_REPRESENTATION_CONTEXT ( 3 ) GLOBAL_UNCERTAINTY_ASSIGNED_CONTEXT ( ( #23172 ) ) GLOBAL_UNIT_ASSIGNED_CONTEXT ( ( #4493, #1128, #6662 ) ) REPRESENTATION_CONTEXT ( 'NONE', 'WORKASPACE' ) );
#13030=CARTESIAN_POINT ( 'NONE',  ( 2.445694354108821411, 2.445694354108820523, 14.31250000136560452 ) ) ;
#13046=VECTOR ( 'NONE', #23596, 1000.000000000000000 ) ;
#13056=CARTESIAN_POINT ( 'NONE',  ( -3.999999999999998224, -1.656854249492383246, 11.06250000000001066 ) ) ;
#13073=CARTESIAN_POINT ( 'NONE',  ( 4.000000000000000888, 4.898587196589412829E-16, 16.62500000273119838 ) ) ;
#13079=CARTESIAN_POINT ( 'NONE',  ( -3.999999999999999112, 0.000000000000000000, 14.00000000000001066 ) ) ;
#13087=EDGE_CURVE ( 'NONE', #5522, #20911, #2846, .T. ) ;
#13091=CARTESIAN_POINT ( 'NONE',  ( -2.445694354108818303, -2.445694354108820523, 15.56250000136560629 ) ) ;
#13096=CARTESIAN_POINT ( 'NONE',  ( -1.432654583217639610, -3.458734124999999882, 11.62500000136560452 ) ) ;
#13104=( BOUNDED_CURVE ( )  B_SPLINE_CURVE ( 2, ( #8119, #5942, #22328, #20883, #10153, #16964, #429, #15546, #893 ),
 .UNSPECIFIED., .F., .F. ) 
 B_SPLINE_CURVE_WITH_KNOTS ( ( 3, 2, 2, 2, 3 ),
 ( 0.5500000000000000444, 0.5625000000000000000, 0.5749999999999999556, 0.5875000000000000222, 0.5999999999999999778 ),
 .UNSPECIFIED. ) 
 CURVE ( )  GEOMETRIC_REPRESENTATION_ITEM ( )  RATIONAL_B_SPLINE_CURVE ( ( 1.000000000000000000, 0.9238795325112867385, 1.000000000000000000, 0.9238795325112867385, 1.000000000000000000, 0.9238795325112867385, 1.000000000000000000, 0.9238795325112867385, 1.000000000000000000 ) ) 
 REPRESENTATION_ITEM ( '' )  );
#13107=ORIENTED_EDGE ( 'NONE', *, *, #5991, .F. ) ;
#13108=CARTESIAN_POINT ( 'NONE',  ( -3.458734124999998993, -1.432654583217642497, 15.75000000136560629 ) ) ;
#13114=CARTESIAN_POINT ( 'NONE',  ( -1.432654583217639166, 3.458734125000000770, 10.50000000136560629 ) ) ;
#13120=CARTESIAN_POINT ( 'NONE',  ( 1.656854249492384135, -3.999999999999999112, 16.43750000273119838 ) ) ;
#13125=ORIENTED_EDGE ( 'NONE', *, *, #14346, .F. ) ;
#13130=VERTEX_POINT ( 'NONE', #14010 ) ;
#13131=CARTESIAN_POINT ( 'NONE',  ( 2.828427124746192067, -2.828427124746189847, 12.37500000000001066 ) ) ;
#13133=LINE ( 'NONE', #20864, #18277 ) ;
#13142=CARTESIAN_POINT ( 'NONE',  ( 3.458734125000001658, 1.432654583217640498, 14.25000000136560629 ) ) ;
#13147=ORIENTED_EDGE ( 'NONE', *, *, #11727, .F. ) ;
#13150=CARTESIAN_POINT ( 'NONE',  ( -20.00000000000000711, 4.500000000000003553, -19.99999999999999645 ) ) ;
#13163=CARTESIAN_POINT ( 'NONE',  ( -3.999999999999999112, -2.265485919601331943, 20.08545885675730602 ) ) ;
#13166=CARTESIAN_POINT ( 'NONE',  ( 1.656854249492384135, -3.999999999999999112, 13.43750000273119838 ) ) ;
#13192=CARTESIAN_POINT ( 'NONE',  ( -3.999999999999999112, 1.656854249492380804, 15.93750000000001066 ) ) ;
#13202=CARTESIAN_POINT ( 'NONE',  ( -1.432654583217639610, -3.458734124999999882, 18.62500000136560274 ) ) ;
#13208=CARTESIAN_POINT ( 'NONE',  ( 3.458734125000001214, 1.432654583217640498, 13.00000000136560452 ) ) ;
#13218=CARTESIAN_POINT ( 'NONE',  ( -20.00000000000001066, 9.999999999999964473, -49.99999999999999289 ) ) ;
#13219=VERTEX_POINT ( 'NONE', #23537 ) ;
#13222=CARTESIAN_POINT ( 'NONE',  ( -1.432654583217639832, -3.458734125000000326, 18.87500000136560274 ) ) ;
#13232=CARTESIAN_POINT ( 'NONE',  ( -0.3649867057748917842, 3.983313282257320509, 9.889028792932920808 ) ) ;
#13236=CARTESIAN_POINT ( 'NONE',  ( 1.971781867644420635E-15, -4.000000000000000000, 15.37500000273119660 ) ) ;
#13237=DIRECTION ( 'NONE',  ( -1.224646799147353207E-16, 0.000000000000000000, -1.000000000000000000 ) ) ;
#13239=DIRECTION ( 'NONE',  ( -0.000000000000000000, -0.000000000000000000, -1.000000000000000000 ) ) ;
#13247=CARTESIAN_POINT ( 'NONE',  ( 4.000000000000000888, 4.898587196589412829E-16, 21.31370849898476649 ) ) ;
#13249=CARTESIAN_POINT ( 'NONE',  ( 2.828427124746191179, 2.828427124746190291, 11.62500000000001066 ) ) ;
#13252=CARTESIAN_POINT ( 'NONE',  ( 4.000000000000000888, 4.898587196589412829E-16, 14.50000000000001066 ) ) ;
#13263=CARTESIAN_POINT ( 'NONE',  ( 3.458734125000001658, 1.432654583217640498, 16.25000000136560629 ) ) ;
#13274=DIRECTION ( 'NONE',  ( -0.000000000000000000, -0.000000000000000000, -1.000000000000000000 ) ) ;
#13285=CARTESIAN_POINT ( 'NONE',  ( -1.656854249492379250, 4.000000000000000000, 12.93750000273119660 ) ) ;
#13306=CARTESIAN_POINT ( 'NONE',  ( -3.999999999999998224, -1.656854249492383246, 13.06250000000001066 ) ) ;
#13321=CARTESIAN_POINT ( 'NONE',  ( -3.458734124999998993, 1.432654583217640276, 13.37500000136560452 ) ) ;
#13340=ORIENTED_EDGE ( 'NONE', *, *, #22661, .F. ) ;
#13341=CARTESIAN_POINT ( 'NONE',  ( 1.025207404391860050E-15, 3.458734125000000770, 17.43750000136560274 ) ) ;
#13344=ADVANCED_FACE ( 'NONE', ( #15293 ), #13374, .T. ) ;
#13356=CARTESIAN_POINT ( 'NONE',  ( -3.999999999999999112, 1.656854249492380804, 17.06250000273120193 ) ) ;
#13359=CARTESIAN_POINT ( 'NONE',  ( 2.828427124746191179, 2.828427124746190291, 13.62500000000001066 ) ) ;
#13360=ORIENTED_EDGE ( 'NONE', *, *, #10568, .F. ) ;
#13365=EDGE_LOOP ( 'NONE', ( #20251, #3377, #4788, #12725 ) ) ;
#13366=CARTESIAN_POINT ( 'NONE',  ( -2.828427124746188515, -2.828427124746190735, 12.12500000000001066 ) ) ;
#13370=ORIENTED_EDGE ( 'NONE', *, *, #9295, .F. ) ;
#13374=CYLINDRICAL_SURFACE ( 'NONE', #13688, 4.000000000000000000 ) ;
#13386=CARTESIAN_POINT ( 'NONE',  ( -2.445694354108818303, -2.445694354108820967, 15.81250000136560629 ) ) ;
#13390=COLOUR_RGB ( '', 0.09019608, 0.27058824, 0.51372549) ;
#13405=LINE ( 'NONE', #20425, #3 ) ;
#13408=ORIENTED_EDGE ( 'NONE', *, *, #10568, .T. ) ;
#13409=CARTESIAN_POINT ( 'NONE',  ( -1.656854249492379250, 4.000000000000000000, 11.93750000273119660 ) ) ;
#13416=VECTOR ( 'NONE', #2029, 1000.000000000000000 ) ;
#13418=VERTEX_POINT ( 'NONE', #4718 ) ;
#13426=CARTESIAN_POINT ( 'NONE',  ( 14.99999999999995559, 15.00000000000000000, -50.00000000000000000 ) ) ;
#13428=VECTOR ( 'NONE', #6977, 1000.000000000000000 ) ;
#13435=CARTESIAN_POINT ( 'NONE',  ( 2.828427124746191179, 2.828427124746190291, 14.62500000000000888 ) ) ;
#13437=ORIENTED_EDGE ( 'NONE', *, *, #3228, .T. ) ;
#13438=DIRECTION ( 'NONE',  ( -1.000000000000000000, 0.000000000000000000, 1.224646799147353207E-16 ) ) ;
#13439=CARTESIAN_POINT ( 'NONE',  ( 9.920644283265380691E-16, 4.000000000000000000, 17.87500000273119483 ) ) ;
#13446=CARTESIAN_POINT ( 'NONE',  ( -1.432654583217638944, 3.458734125000000326, 14.25000000136560629 ) ) ;
#13465=CARTESIAN_POINT ( 'NONE',  ( -3.458734124999999437, 1.432654583217640498, 15.62500000136560629 ) ) ;
#13476=CARTESIAN_POINT ( 'NONE',  ( 4.000000000000000888, 4.898587196589412829E-16, 10.62500000273119660 ) ) ;
#13487=CARTESIAN_POINT ( 'NONE',  ( 4.000000000000000888, 4.898587196589412829E-16, 12.50000000000001066 ) ) ;
#13492=EDGE_CURVE ( 'NONE', #17728, #19630, #5069, .T. ) ;
#13495=CARTESIAN_POINT ( 'NONE',  ( 1.971781867644420635E-15, -4.000000000000000000, 15.25000000000001066 ) ) ;
#13496=CARTESIAN_POINT ( 'NONE',  ( -2.445694354108819191, 2.445694354108820523, 19.56250000136560629 ) ) ;
#13502=CARTESIAN_POINT ( 'NONE',  ( 2.445694354108822299, -2.445694354108820079, 11.06250000136560452 ) ) ;
#13512=VERTEX_POINT ( 'NONE', #17886 ) ;
#13528=DIRECTION ( 'NONE',  ( 0.000000000000000000, -0.000000000000000000, -1.000000000000000000 ) ) ;
#13543=CARTESIAN_POINT ( 'NONE',  ( -3.999999999999999112, 1.656854249492380804, 10.93750000000001421 ) ) ;
#13552=CARTESIAN_POINT ( 'NONE',  ( 35.00000000000000000, 7.500000000000001776, -20.00000000000000355 ) ) ;
#13554=CARTESIAN_POINT ( 'NONE',  ( 2.445694354108821855, -2.445694354108820079, 13.81250000136560629 ) ) ;
#13560=CARTESIAN_POINT ( 'NONE',  ( -3.458734124999998993, 0.000000000000000000, 11.43750000136560452 ) ) ;
#13571=CARTESIAN_POINT ( 'NONE',  ( 3.458734125000002546, -1.432654583217639610, 17.12500000136560629 ) ) ;
#13577=AXIS2_PLACEMENT_3D ( 'NONE', #19652, #3253, #12274 ) ;
#13585=CARTESIAN_POINT ( 'NONE',  ( 2.828427124746192067, -2.828427124746189847, 10.50000000273119660 ) ) ;
#13597=CARTESIAN_POINT ( 'NONE',  ( -3.999999999999999112, 1.656854249492380804, 14.93750000000000888 ) ) ;
#13605=CYLINDRICAL_SURFACE ( 'NONE', #23280, 4.000000000000000000 ) ;
#13615=CARTESIAN_POINT ( 'NONE',  ( 1.432654583217643163, -3.458734124999999882, 11.00000000136560452 ) ) ;
#13624=ORIENTED_EDGE ( 'NONE', *, *, #1236, .F. ) ;
#13639=CARTESIAN_POINT ( 'NONE',  ( -3.999999999999998224, -1.656854249492383024, 12.18750000273119838 ) ) ;
#13657=ORIENTED_EDGE ( 'NONE', *, *, #11168, .F. ) ;
#13662=CARTESIAN_POINT ( 'NONE',  ( 14.99999999999999289, -10.00000000000000000, -50.00000000000000000 ) ) ;
#13665=VERTEX_POINT ( 'NONE', #587 ) ;
#13667=EDGE_CURVE ( 'NONE', #12476, #1631, #1587, .T. ) ;
#13671=CARTESIAN_POINT ( 'NONE',  ( 1.432654583217643163, -3.458734124999999437, 12.75000000136560629 ) ) ;
#13674=CARTESIAN_POINT ( 'NONE',  ( 34.99999999999999289, 4.500000000000001776, -50.00000000000000000 ) ) ;
#13688=AXIS2_PLACEMENT_3D ( 'NONE', #20643, #878, #18851 ) ;
#13690=CARTESIAN_POINT ( 'NONE',  ( 1.432654583217643163, -3.458734124999999882, 12.00000000136560452 ) ) ;
#13703=CARTESIAN_POINT ( 'NONE',  ( -3.999999999999998224, -1.656854249492383246, 10.18750000273119660 ) ) ;
#13708=CARTESIAN_POINT ( 'NONE',  ( -3.999999999999999112, 0.000000000000000000, 17.12500000273119838 ) ) ;
#13727=CARTESIAN_POINT ( 'NONE',  ( 2.445694354108821411, 2.445694354108820523, 19.31250000136560629 ) ) ;
#13733=CARTESIAN_POINT ( 'NONE',  ( -1.432654583217639166, 3.458734125000000770, 11.50000000136560629 ) ) ;
#13743=ORIENTED_EDGE ( 'NONE', *, *, #7439, .F. ) ;
#13749=VERTEX_POINT ( 'NONE', #17127 ) ;
#13763=DIRECTION ( 'NONE',  ( 1.000000000000000000, 0.000000000000000000, -0.000000000000000000 ) ) ;
#13768=EDGE_LOOP ( 'NONE', ( #2988, #12083, #11044, #767 ) ) ;
#13797=CARTESIAN_POINT ( 'NONE',  ( -3.458734124999998993, -1.432654583217642497, 12.50000000136560452 ) ) ;
#13802=ORIENTED_EDGE ( 'NONE', *, *, #2597, .F. ) ;
#13817=CARTESIAN_POINT ( 'NONE',  ( -3.458734124999999437, 0.000000000000000000, 12.68750000136560629 ) ) ;
#13819=VECTOR ( 'NONE', #11166, 1000.000000000000000 ) ;
#13820=EDGE_CURVE ( 'NONE', #11553, #4495, #19028, .T. ) ;
#13827=DIRECTION ( 'NONE',  ( 1.000000000000000000, 0.000000000000000000, -1.224646799147353207E-16 ) ) ;
#13831=CARTESIAN_POINT ( 'NONE',  ( -3.999999999999999112, 0.000000000000000000, 13.12500000273119660 ) ) ;
#13835=CARTESIAN_POINT ( 'NONE',  ( 14.99999999999999289, -10.00000000000000000, -50.00000000000000000 ) ) ;
#13836=ORIENTED_EDGE ( 'NONE', *, *, #8605, .T. ) ;
#13851=CARTESIAN_POINT ( 'NONE',  ( 9.920644283265380691E-16, 4.000000000000000000, 14.87500000273119660 ) ) ;
#13854=PLANE ( 'NONE',  #3061 ) ;
#13869=( BOUNDED_CURVE ( )  B_SPLINE_CURVE ( 2, ( #4651, #2487, #4299 ),
 .UNSPECIFIED., .F., .F. ) 
 B_SPLINE_CURVE_WITH_KNOTS ( ( 3, 3 ),
 ( 0.9155333511103322941, 0.9235200992307018852 ),
 .UNSPECIFIED. ) 
 CURVE ( )  GEOMETRIC_REPRESENTATION_ITEM ( )  RATIONAL_B_SPLINE_CURVE ( ( 0.9720211172018224932, 0.9469897216464003842, 0.9841097943611590848 ) ) 
 REPRESENTATION_ITEM ( '' )  );
#13873=UNCERTAINTY_MEASURE_WITH_UNIT (LENGTH_MEASURE( 1.000000000000000082E-05 ), #7380, 'distance_accuracy_value', 'NONE');
#13878=DIRECTION ( 'NONE',  ( -1.000000000000000000, 0.000000000000000000, 0.000000000000000000 ) ) ;
#13881=CARTESIAN_POINT ( 'NONE',  ( -1.432654583217638944, 3.458734125000000326, 17.25000000136560274 ) ) ;
#13884=ORIENTED_EDGE ( 'NONE', *, *, #13820, .T. ) ;
#13906=DIRECTION ( 'NONE',  ( -1.224646799147353207E-16, 0.000000000000000000, -1.000000000000000000 ) ) ;
#13908=CARTESIAN_POINT ( 'NONE',  ( -3.458734124999999437, 1.432654583217640498, 19.62500000136560629 ) ) ;
#13910=AXIS2_PLACEMENT_3D ( 'NONE', #15599, #1293, #1409 ) ;
#13918=EDGE_CURVE ( 'NONE', #18283, #7307, #11699, .T. ) ;
#13920=CARTESIAN_POINT ( 'NONE',  ( 1.656854249492384135, -3.999999999999999112, 13.43750000273119838 ) ) ;
#13926=VERTEX_POINT ( 'NONE', #21271 ) ;
#13928=CARTESIAN_POINT ( 'NONE',  ( -1.432654583217639832, -3.458734125000000326, 12.87500000136560629 ) ) ;
#13929=LINE ( 'NONE', #8536, #14968 ) ;
#13941=CARTESIAN_POINT ( 'NONE',  ( 4.000000000000000888, 4.898587196589412829E-16, 11.62500000273119660 ) ) ;
#13946=CARTESIAN_POINT ( 'NONE',  ( 0.9413949561959078505, 0.3373062947069096484, 10.00000000000000888 ) ) ;
#13954=CARTESIAN_POINT ( 'NONE',  ( -3.999999999999999112, 0.000000000000000000, 20.00000000000001066 ) ) ;
#13960=CARTESIAN_POINT ( 'NONE',  ( -2.445694354108819191, 2.445694354108820523, 17.56250000136560274 ) ) ;
#13961=CARTESIAN_POINT ( 'NONE',  ( -3.999999999999999112, 1.656854249492380804, 14.06250000273119660 ) ) ;
#13987=CYLINDRICAL_SURFACE ( 'NONE', #2817, 4.000000000000000000 ) ;
#13991=CARTESIAN_POINT ( 'NONE',  ( 2.445694354108821855, -2.445694354108820079, 14.81250000136560452 ) ) ;
#13996=( BOUNDED_CURVE ( )  B_SPLINE_CURVE ( 2, ( #22733, #21154, #10314, #17602, #19019, #4655, #1049, #2491, #6345 ),
 .UNSPECIFIED., .F., .F. ) 
 B_SPLINE_CURVE_WITH_KNOTS ( ( 3, 2, 2, 2, 3 ),
 ( 0.2000000000000000111, 0.2124999999999999944, 0.2250000000000000056, 0.2374999999999999889, 0.2500000000000000000 ),
 .UNSPECIFIED. ) 
 CURVE ( )  GEOMETRIC_REPRESENTATION_ITEM ( )  RATIONAL_B_SPLINE_CURVE ( ( 1.000000000000000000, 0.9238795325112867385, 1.000000000000000000, 0.9238795325112867385, 1.000000000000000000, 0.9238795325112867385, 1.000000000000000000, 0.9238795325112867385, 1.000000000000000000 ) ) 
 REPRESENTATION_ITEM ( '' )  );
#14010=CARTESIAN_POINT ( 'NONE',  ( -3.999999999999999112, 0.000000000000000000, 13.00000000000001066 ) ) ;
#14012=CARTESIAN_POINT ( 'NONE',  ( 4.000000000000000888, 4.898587196589412829E-16, 11.50000000000001066 ) ) ;
#14018=CARTESIAN_POINT ( 'NONE',  ( -3.458734124999998993, -1.432654583217642497, 18.75000000136560274 ) ) ;
#14023=CARTESIAN_POINT ( 'NONE',  ( -3.999999999999999112, 0.000000000000000000, 16.00000000000001066 ) ) ;
#14032=ADVANCED_FACE ( 'NONE', ( #3453 ), #16506, .T. ) ;
#14035=CARTESIAN_POINT ( 'NONE',  ( 1.025207404391860050E-15, 3.458734125000000770, 12.43750000136560629 ) ) ;
#14045=CARTESIAN_POINT ( 'NONE',  ( 2.828427124746192067, -2.828427124746189847, 13.37500000000001243 ) ) ;
#14046=CARTESIAN_POINT ( 'NONE',  ( 34.99999999999999289, 7.500000000000001776, -50.00000000000000000 ) ) ;
#14047=CARTESIAN_POINT ( 'NONE',  ( 3.458734125000002102, -1.432654583217639610, 15.87500000136560807 ) ) ;
#14050=CARTESIAN_POINT ( 'NONE',  ( -1.656854249492380138, -3.999999999999999112, 14.31250000273119660 ) ) ;
#14051=ORIENTED_EDGE ( 'NONE', *, *, #9186, .T. ) ;
#14064=LINE ( 'NONE', #12398, #10297 ) ;
#14075=CARTESIAN_POINT ( 'NONE',  ( -2.445694354108819191, 2.445694354108820523, 14.56250000136560452 ) ) ;
#14076=CARTESIAN_POINT ( 'NONE',  ( 4.000000000000000888, 4.898587196589412829E-16, 10.62500000273119660 ) ) ;
#14082=CARTESIAN_POINT ( 'NONE',  ( 1.656854249492384135, -3.999999999999999112, 18.43750000273119483 ) ) ;
#14087=ORIENTED_EDGE ( 'NONE', *, *, #12662, .T. ) ;
#14097=FILL_AREA_STYLE ('',( #21362 ) ) ;
#14101=CARTESIAN_POINT ( 'NONE',  ( 4.000000000000001776, -1.656854249492379694, 11.43750000000001066 ) ) ;
#14108=CARTESIAN_POINT ( 'NONE',  ( 4.000000000000000888, 4.898587196589412829E-16, 17.62500000273119483 ) ) ;
#14113=CARTESIAN_POINT ( 'NONE',  ( -1.432654583217639610, -3.458734124999999882, 14.62500000136560452 ) ) ;
#14116=FACE_OUTER_BOUND ( 'NONE', #20027, .T. ) ;
#14128=ORIENTED_EDGE ( 'NONE', *, *, #22864, .F. ) ;
#14133=CARTESIAN_POINT ( 'NONE',  ( 1.656854249492384135, -3.999999999999999112, 16.31250000000001066 ) ) ;
#14136=VERTEX_POINT ( 'NONE', #23036 ) ;
#14141=CARTESIAN_POINT ( 'NONE',  ( 2.445694354108821411, 2.445694354108820523, 19.31250000136560629 ) ) ;
#14149=DIRECTION ( 'NONE',  ( -1.224646799147353207E-16, 0.000000000000000000, -1.000000000000000000 ) ) ;
#14156=VECTOR ( 'NONE', #5336, 1000.000000000000000 ) ;
#14162=CARTESIAN_POINT ( 'NONE',  ( 1.025207404391860050E-15, 3.458734125000000770, 14.43750000136560452 ) ) ;
#14164=LINE ( 'NONE', #18208, #13046 ) ;
#14176=CARTESIAN_POINT ( 'NONE',  ( -2.247776618166700491, 3.308700692843503877, 10.00000000000000888 ) ) ;
#14177=CARTESIAN_POINT ( 'NONE',  ( -2.445694354108819191, 2.445694354108820523, 16.31250000136560629 ) ) ;
#14178=LINE ( 'NONE', #12385, #13428 ) ;
#14199=CARTESIAN_POINT ( 'NONE',  ( 3.458734125000002546, -1.432654583217639610, 14.12500000136560452 ) ) ;
#14206=EDGE_CURVE ( 'NONE', #16922, #10607, #5094, .T. ) ;
#14209=DIRECTION ( 'NONE',  ( -1.734723475976805517E-15, 0.000000000000000000, 1.000000000000000000 ) ) ;
#14221=ORIENTED_EDGE ( 'NONE', *, *, #784, .F. ) ;
#14227=CARTESIAN_POINT ( 'NONE',  ( 9.920644283265380691E-16, 4.000000000000000000, 10.75000000000001066 ) ) ;
#14232=CARTESIAN_POINT ( 'NONE',  ( 27.50000000000000000, 4.500000000000001776, -31.01025403784447221 ) ) ;
#14235=EDGE_CURVE ( 'NONE', #14480, #8531, #18087, .T. ) ;
#14238=CARTESIAN_POINT ( 'NONE',  ( -2.445694354108818303, -2.445694354108820523, 16.56250000136560629 ) ) ;
#14260=CARTESIAN_POINT ( 'NONE',  ( -3.999999999999999112, 1.656854249492380582, 10.06250000273119660 ) ) ;
#14262=DIRECTION ( 'NONE',  ( 0.000000000000000000, 1.000000000000000000, 0.000000000000000000 ) ) ;
#14264=CARTESIAN_POINT ( 'NONE',  ( -3.458734124999998993, -1.432654583217642497, 17.75000000136560629 ) ) ;
#14270=CARTESIAN_POINT ( 'NONE',  ( -2.828427124746189403, 2.828427124746190291, 11.00000000273119660 ) ) ;
#14272=EDGE_CURVE ( 'NONE', #22281, #12677, #8327, .T. ) ;
#14282=CARTESIAN_POINT ( 'NONE',  ( -1.656854249492379250, 4.000000000000000000, 19.81250000000001776 ) ) ;
#14294=CARTESIAN_POINT ( 'NONE',  ( -1.432654583217639610, -3.458734124999999882, 17.62500000136560274 ) ) ;
#14297=FACE_OUTER_BOUND ( 'NONE', #8057, .T. ) ;
#14316=CARTESIAN_POINT ( 'NONE',  ( 1.872352939448454495E-15, -3.458734125000000770, 16.93750000136560629 ) ) ;
#14332=CARTESIAN_POINT ( 'NONE',  ( 1.656854249492384135, -3.999999999999999112, 16.31250000000001066 ) ) ;
#14341=CARTESIAN_POINT ( 'NONE',  ( 4.000000000000000888, 4.898587196589412829E-16, 11.50000000000001066 ) ) ;
#14346=EDGE_CURVE ( 'NONE', #10762, #839, #18111, .T. ) ;
#14353=CARTESIAN_POINT ( 'NONE',  ( 3.458734125000002102, -1.432654583217639610, 15.87500000136560452 ) ) ;
#14354=CARTESIAN_POINT ( 'NONE',  ( 1.656854249492384135, -3.999999999999999112, 18.43750000273119483 ) ) ;
#14362=EDGE_CURVE ( 'NONE', #12919, #8667, #5656, .T. ) ;
#14367=ORIENTED_EDGE ( 'NONE', *, *, #18879, .F. ) ;
#14383=PLANE ( 'NONE',  #22525 ) ;
#14386=DIRECTION ( 'NONE',  ( 0.000000000000000000, -1.000000000000000000, 0.000000000000000000 ) ) ;
#14399=CARTESIAN_POINT ( 'NONE',  ( -1.656854249492379472, 4.000000000000000000, 18.81250000000001421 ) ) ;
#14400=CARTESIAN_POINT ( 'NONE',  ( -1.656854249492379250, 4.000000000000000000, 18.81250000000001776 ) ) ;
#14416=CARTESIAN_POINT ( 'NONE',  ( 1.432654583217641164, 3.458734125000000326, 17.12500000136560629 ) ) ;
#14433=CARTESIAN_POINT ( 'NONE',  ( 1.432654583217641386, 3.458734125000000770, 16.37500000136560629 ) ) ;
#14439=CARTESIAN_POINT ( 'NONE',  ( -3.999999999999999112, 1.656854249492380804, 18.06250000273119838 ) ) ;
#14442=EDGE_CURVE ( 'NONE', #14730, #315, #18437, .T. ) ;
#14449=DIRECTION ( 'NONE',  ( -0.000000000000000000, 1.000000000000000000, -0.000000000000000000 ) ) ;
#14451=CARTESIAN_POINT ( 'NONE',  ( -1.656854249492379250, 4.000000000000000000, 16.81250000000001066 ) ) ;
#14456=FACE_BOUND ( 'NONE', #18203, .T. ) ;
#14469=CARTESIAN_POINT ( 'NONE',  ( -3.458734124999998993, 0.000000000000000000, 13.43750000136560452 ) ) ;
#14480=VERTEX_POINT ( 'NONE', #7440 ) ;
#14484=EDGE_CURVE ( 'NONE', #11306, #4949, #6646, .T. ) ;
#14487=DIRECTION ( 'NONE',  ( -0.000000000000000000, -1.000000000000000000, 0.000000000000000000 ) ) ;
#14497=CARTESIAN_POINT ( 'NONE',  ( 9.920644283265380691E-16, 4.000000000000000000, 10.75000000000001066 ) ) ;
#14505=DIRECTION ( 'NONE',  ( -1.000000000000000000, 0.000000000000000000, 1.224646799147353207E-16 ) ) ;
#14522=CARTESIAN_POINT ( 'NONE',  ( -3.999999999999999112, 0.000000000000000000, 19.00000000000001066 ) ) ;
#14524=CARTESIAN_POINT ( 'NONE',  ( -3.458734124999999437, 1.432654583217640498, 10.62500000136560452 ) ) ;
#14526=DIRECTION ( 'NONE',  ( 0.000000000000000000, 0.000000000000000000, 1.000000000000000000 ) ) ;
#14528=AXIS2_PLACEMENT_3D ( 'NONE', #4194, #4311, #9720 ) ;
#14529=DIRECTION ( 'NONE',  ( -1.000000000000000000, 0.000000000000000000, 0.000000000000000000 ) ) ;
#14533=CARTESIAN_POINT ( 'NONE',  ( -3.458734124999998993, -1.432654583217642497, 17.50000000136560274 ) ) ;
#14535=PRODUCT_DEFINITION_FORMATION_WITH_SPECIFIED_SOURCE ( 'ANY', '', #11660, .NOT_KNOWN. ) ;
#14539=ADVANCED_FACE ( 'NONE', ( #20455 ), #9602, .F. ) ;
#14541=CARTESIAN_POINT ( 'NONE',  ( 1.432654583217641164, 3.458734125000000326, 19.12500000136560629 ) ) ;
#14545=ORIENTED_EDGE ( 'NONE', *, *, #8605, .F. ) ;
#14553=VECTOR ( 'NONE', #1505, 1000.000000000000000 ) ;
#14560=CARTESIAN_POINT ( 'NONE',  ( 3.458734125000001658, 1.432654583217640498, 11.25000000136560452 ) ) ;
#14561=CARTESIAN_POINT ( 'NONE',  ( -2.828427124746188515, -2.828427124746190735, 11.25000000273119660 ) ) ;
#14569=CIRCLE ( 'NONE', #16077, 4.000000000000000888 ) ;
#14577=EDGE_CURVE ( 'NONE', #21889, #12232, #13996, .T. ) ;
#14580=CARTESIAN_POINT ( 'NONE',  ( 2.828427124746192067, -2.828427124746189847, 17.37500000000001066 ) ) ;
#14584=ORIENTED_EDGE ( 'NONE', *, *, #11168, .T. ) ;
#14585=DIRECTION ( 'NONE',  ( 0.000000000000000000, -1.000000000000000000, 0.000000000000000000 ) ) ;
#14586=CYLINDRICAL_SURFACE ( 'NONE', #1791, 4.000000000000000000 ) ;
#14597=VERTEX_POINT ( 'NONE', #19145 ) ;
#14599=CARTESIAN_POINT ( 'NONE',  ( -3.999999999999999112, 0.000000000000000000, 11.12500000273119660 ) ) ;
#14616=CARTESIAN_POINT ( 'NONE',  ( -2.828427124746189403, 2.828427124746190291, 18.00000000273119483 ) ) ;
#14627=CARTESIAN_POINT ( 'NONE',  ( -3.999999999999999112, 0.000000000000000000, 17.00000000000001066 ) ) ;
#14629=VERTEX_POINT ( 'NONE', #12104 ) ;
#14633=VERTEX_POINT ( 'NONE', #1167 ) ;
#14638=CARTESIAN_POINT ( 'NONE',  ( 1.656854249492384135, -3.999999999999999112, 17.31250000000001421 ) ) ;
#14648=ADVANCED_FACE ( 'NONE', ( #4578, #6615 ), #17515, .T. ) ;
#14650=CARTESIAN_POINT ( 'NONE',  ( 2.445694354108821411, 2.445694354108820523, 19.06250000136560629 ) ) ;
#14654=CARTESIAN_POINT ( 'NONE',  ( 1.872352939448454495E-15, -3.458734125000000326, 13.68750000136560629 ) ) ;
#14672=CARTESIAN_POINT ( 'NONE',  ( 2.445694354108821411, 2.445694354108820523, 11.31250000136560452 ) ) ;
#14677=ADVANCED_FACE ( 'NONE', ( #21303 ), #2997, .T. ) ;
#14678=APPLICATION_CONTEXT ( 'automotive_design' ) ;
#14680=CARTESIAN_POINT ( 'NONE',  ( -3.999999999999998224, -1.656854249492383246, 17.18750000273119838 ) ) ;
#14681=DIRECTION ( 'NONE',  ( -0.000000000000000000, 1.000000000000000000, -0.000000000000000000 ) ) ;
#14682=AXIS2_PLACEMENT_3D ( 'NONE', #23583, #1656, #3685 ) ;
#14692=CARTESIAN_POINT ( 'NONE',  ( 4.000000000000000888, 1.656854249492381248, 15.56250000000000888 ) ) ;
#14704=ADVANCED_FACE ( 'NONE', ( #15497 ), #11171, .T. ) ;
#14708=CARTESIAN_POINT ( 'NONE',  ( 3.458734125000001658, 1.432654583217640498, 19.25000000136560274 ) ) ;
#14711=CARTESIAN_POINT ( 'NONE',  ( -3.999999999999999112, 0.000000000000000000, 17.00000000000001066 ) ) ;
#14720=ORIENTED_EDGE ( 'NONE', *, *, #21094, .F. ) ;
#14721=DIRECTION ( 'NONE',  ( 0.000000000000000000, 0.000000000000000000, -1.000000000000000000 ) ) ;
#14730=VERTEX_POINT ( 'NONE', #19988 ) ;
#14731=CARTESIAN_POINT ( 'NONE',  ( 1.656854249492381470, 4.000000000000000000, 16.81250000273119838 ) ) ;
#14739=FACE_OUTER_BOUND ( 'NONE', #23385, .T. ) ;
#14749=CIRCLE ( 'NONE', #9370, 4.999999999999999112 ) ;
#14752=ORIENTED_EDGE ( 'NONE', *, *, #3363, .F. ) ;
#14755=CARTESIAN_POINT ( 'NONE',  ( -3.458734124999998993, -1.432654583217642497, 10.75000000136560452 ) ) ;
#14760=ORIENTED_EDGE ( 'NONE', *, *, #1937, .T. ) ;
#14767=CARTESIAN_POINT ( 'NONE',  ( -1.432654583217638944, 3.458734125000000326, 19.25000000136560274 ) ) ;
#14770=CARTESIAN_POINT ( 'NONE',  ( 4.000000000000000888, 4.898587196589412829E-16, 12.50000000000001066 ) ) ;
#14771=CARTESIAN_POINT ( 'NONE',  ( 3.458734125000001214, 1.432654583217640498, 12.00000000136560452 ) ) ;
#14781=EDGE_CURVE ( 'NONE', #1631, #12232, #3483, .T. ) ;
#14788=CARTESIAN_POINT ( 'NONE',  ( 3.458734125000002546, -1.432654583217639610, 19.12500000136560629 ) ) ;
#14799=CARTESIAN_POINT ( 'NONE',  ( 4.000000000000000888, 1.656854249492381248, 15.68750000273119660 ) ) ;
#14811=CARTESIAN_POINT ( 'NONE',  ( -1.656854249492379250, 4.000000000000000000, 15.81250000000001066 ) ) ;
#14824=CARTESIAN_POINT ( 'NONE',  ( 1.025207404391860050E-15, 3.458734125000000770, 14.43750000136560452 ) ) ;
#14827=CARTESIAN_POINT ( 'NONE',  ( -1.656854249492379472, 4.000000000000000000, 16.81250000000001066 ) ) ;
#14839=CARTESIAN_POINT ( 'NONE',  ( -3.999999999999998224, -1.656854249492383024, 18.06250000000001421 ) ) ;
#14849=CARTESIAN_POINT ( 'NONE',  ( 1.656854249492381470, 4.000000000000000000, 17.81250000273119483 ) ) ;
#14857=AXIS2_PLACEMENT_3D ( 'NONE', #5061, #6986, #7790 ) ;
#14870=ORIENTED_EDGE ( 'NONE', *, *, #4248, .F. ) ;
#14871=DIRECTION ( 'NONE',  ( -1.000000000000000000, 0.000000000000000000, 1.224646799147353207E-16 ) ) ;
#14875=CARTESIAN_POINT ( 'NONE',  ( -2.828427124746188515, -2.828427124746190735, 16.12500000000001066 ) ) ;
#14881=CARTESIAN_POINT ( 'NONE',  ( 4.000000000000000888, 4.898587196589412829E-16, 17.62500000273119483 ) ) ;
#14887=CARTESIAN_POINT ( 'NONE',  ( 2.445694354108821411, 2.445694354108820523, 16.06250000136560629 ) ) ;
#14892=CARTESIAN_POINT ( 'NONE',  ( 3.458734125000001214, 4.235727675282971730E-16, 12.93750000136560452 ) ) ;
#14904=VERTEX_POINT ( 'NONE', #18066 ) ;
#14905=CARTESIAN_POINT ( 'NONE',  ( 1.432654583217643163, -3.458734124999999882, 16.00000000136560629 ) ) ;
#14910=EDGE_CURVE ( 'NONE', #13512, #13219, #1762, .T. ) ;
#14913=CARTESIAN_POINT ( 'NONE',  ( -1.432654583217639166, 3.458734125000000770, 11.50000000136560452 ) ) ;
#14918=( BOUNDED_CURVE ( )  B_SPLINE_CURVE ( 2, ( #2953, #10307, #15804, #5358, #8607, #8980, #1518, #23676, #1270 ),
 .UNSPECIFIED., .F., .F. ) 
 B_SPLINE_CURVE_WITH_KNOTS ( ( 3, 2, 2, 2, 3 ),
 ( 0.5000000000000000000, 0.5124999999999999556, 0.5250000000000000222, 0.5374999999999999778, 0.5500000000000000444 ),
 .UNSPECIFIED. ) 
 CURVE ( )  GEOMETRIC_REPRESENTATION_ITEM ( )  RATIONAL_B_SPLINE_CURVE ( ( 1.000000000000000000, 0.9238795325112867385, 1.000000000000000000, 0.9238795325112867385, 1.000000000000000000, 0.9238795325112867385, 1.000000000000000000, 0.9238795325112867385, 1.000000000000000000 ) ) 
 REPRESENTATION_ITEM ( '' )  );
#14920=CARTESIAN_POINT ( 'NONE',  ( -3.458734124999998993, 0.000000000000000000, 11.43750000136560452 ) ) ;
#14922=CARTESIAN_POINT ( 'NONE',  ( -1.656854249492380138, -3.999999999999999112, 15.31250000273119660 ) ) ;
#14927=ORIENTED_EDGE ( 'NONE', *, *, #6597, .T. ) ;
#14930=EDGE_LOOP ( 'NONE', ( #18961, #2946, #11504, #23281 ) ) ;
#14935=CARTESIAN_POINT ( 'NONE',  ( -3.999999999999999112, 0.000000000000000000, 13.00000000000001066 ) ) ;
#14937=CIRCLE ( 'NONE', #385, 4.999999999999999112 ) ;
#14952=CARTESIAN_POINT ( 'NONE',  ( 3.458734125000001658, 1.432654583217640498, 15.25000000136560807 ) ) ;
#14966=CARTESIAN_POINT ( 'NONE',  ( 1.656854249492384135, -3.999999999999999112, 18.31250000000001421 ) ) ;
#14968=VECTOR ( 'NONE', #21183, 1000.000000000000000 ) ;
#14976=ADVANCED_FACE ( 'NONE', ( #2551 ), #13605, .T. ) ;
#14978=CARTESIAN_POINT ( 'NONE',  ( -3.999999999999999112, 1.656854249492380804, 18.06250000273119838 ) ) ;
#14984=VECTOR ( 'NONE', #16515, 1000.000000000000000 ) ;
#15002=CARTESIAN_POINT ( 'NONE',  ( -1.656854249492380138, -3.999999999999999112, 15.18750000000001066 ) ) ;
#15011=CARTESIAN_POINT ( 'NONE',  ( 1.432654583217643163, -3.458734124999999437, 18.75000000136560274 ) ) ;
#15017=CARTESIAN_POINT ( 'NONE',  ( -1.432654583217638944, 3.458734125000000326, 14.25000000136560629 ) ) ;
#15028=CARTESIAN_POINT ( 'NONE',  ( 1.432654583217643163, -3.458734124999999882, 18.00000000136560274 ) ) ;
#15033=CARTESIAN_POINT ( 'NONE',  ( -3.458734124999999437, 1.432654583217640498, 11.62500000136560629 ) ) ;
#15034=DIRECTION ( 'NONE',  ( 1.224646799147353207E-16, -0.000000000000000000, 1.000000000000000000 ) ) ;
#15039=CARTESIAN_POINT ( 'NONE',  ( -2.828427124746189403, 2.828427124746190291, 16.00000000273119838 ) ) ;
#15040=CARTESIAN_POINT ( 'NONE',  ( 9.920644283265380691E-16, 4.000000000000000000, 10.75000000000001066 ) ) ;
#15041=ORIENTED_EDGE ( 'NONE', *, *, #19346, .F. ) ;
#15052=CARTESIAN_POINT ( 'NONE',  ( 9.920644283265380691E-16, 4.000000000000000000, 11.75000000000001066 ) ) ;
#15055=CARTESIAN_POINT ( 'NONE',  ( -1.656854249492379472, 4.000000000000000000, 14.81250000000000888 ) ) ;
#15061=CARTESIAN_POINT ( 'NONE',  ( 1.971781867644420635E-15, -4.000000000000000000, 11.25000000000001066 ) ) ;
#15066=CARTESIAN_POINT ( 'NONE',  ( 3.458734125000002546, -1.432654583217639610, 13.12500000136560629 ) ) ;
#15085=EDGE_CURVE ( 'NONE', #17303, #8531, #23630, .T. ) ;
#15090=ORIENTED_EDGE ( 'NONE', *, *, #11992, .T. ) ;
#15091=CARTESIAN_POINT ( 'NONE',  ( 1.971781867644420635E-15, -4.000000000000000000, 15.37500000273119660 ) ) ;
#15094=FACE_OUTER_BOUND ( 'NONE', #6782, .T. ) ;
#15101=ADVANCED_FACE ( 'NONE', ( #22796 ), #6408, .T. ) ;
#15107=CARTESIAN_POINT ( 'NONE',  ( -3.999999999999999112, 0.000000000000000000, 16.12500000273119838 ) ) ;
#15109=DIRECTION ( 'NONE',  ( -0.000000000000000000, -0.000000000000000000, -1.000000000000000000 ) ) ;
#15111=CARTESIAN_POINT ( 'NONE',  ( -2.828427124746188515, -2.828427124746190735, 14.12500000000001066 ) ) ;
#15122=CARTESIAN_POINT ( 'NONE',  ( -3.458734124999998993, 0.000000000000000000, 14.43750000136560452 ) ) ;
#15129=CARTESIAN_POINT ( 'NONE',  ( -3.458734124999998993, 0.000000000000000000, 15.43750000136560452 ) ) ;
#15132=CARTESIAN_POINT ( 'NONE',  ( 4.000000000000000888, 1.656854249492381248, 15.68750000273119660 ) ) ;
#15141=CARTESIAN_POINT ( 'NONE',  ( -1.432654583217639166, 3.458734125000000770, 18.50000000136560629 ) ) ;
#15154=CARTESIAN_POINT ( 'NONE',  ( -2.445694354108818303, -2.445694354108820523, 11.56250000136560629 ) ) ;
#15155=CARTESIAN_POINT ( 'NONE',  ( -2.828427124746188515, -2.828427124746190735, 14.25000000273119660 ) ) ;
#15167=CARTESIAN_POINT ( 'NONE',  ( 9.920644283265380691E-16, 4.000000000000000000, 12.75000000000001066 ) ) ;
#15170=CARTESIAN_POINT ( 'NONE',  ( -20.00000000000001066, -10.00000000000000000, -49.99999999999999289 ) ) ;
#15182=CARTESIAN_POINT ( 'NONE',  ( -3.458734124999998993, -1.432654583217642497, 15.75000000136560629 ) ) ;
#15197=CARTESIAN_POINT ( 'NONE',  ( -1.656854249492379250, 4.000000000000000000, 19.81250000000001776 ) ) ;
#15200=CARTESIAN_POINT ( 'NONE',  ( -3.999999999999999112, 0.000000000000000000, 12.12500000273119838 ) ) ;
#15206=CARTESIAN_POINT ( 'NONE',  ( 3.458734125000001214, 4.235727675282971730E-16, 16.93750000136560629 ) ) ;
#15210=CARTESIAN_POINT ( 'NONE',  ( 35.00000000000000000, 7.500000000000001776, -20.00000000000000355 ) ) ;
#15225=CARTESIAN_POINT ( 'NONE',  ( 1.656854249492381470, 4.000000000000000000, 12.68750000000001243 ) ) ;
#15239=CARTESIAN_POINT ( 'NONE',  ( -3.458734124999998993, 1.432654583217640276, 12.37500000136560629 ) ) ;
#15260=CARTESIAN_POINT ( 'NONE',  ( 1.872352939448454495E-15, -3.458734125000000770, 17.93750000136560274 ) ) ;
#15273=CARTESIAN_POINT ( 'NONE',  ( 1.432654583217643163, -3.458734124999999437, 12.75000000136560629 ) ) ;
#15274=CARTESIAN_POINT ( 'NONE',  ( 1.656854249492381470, 4.000000000000000000, 10.81250000273119660 ) ) ;
#15285=CARTESIAN_POINT ( 'NONE',  ( -2.828427124746188515, -2.828427124746190735, 15.12500000000001066 ) ) ;
#15293=FACE_OUTER_BOUND ( 'NONE', #3947, .T. ) ;
#15295=CARTESIAN_POINT ( 'NONE',  ( -1.656854249492380138, -3.999999999999999112, 15.18750000000001066 ) ) ;
#15304=CARTESIAN_POINT ( 'NONE',  ( 1.025207404391860050E-15, 3.458734125000000770, 16.43750000136560629 ) ) ;
#15331=CARTESIAN_POINT ( 'NONE',  ( 2.828427124746192067, -2.828427124746189847, 12.50000000273119838 ) ) ;
#15332=CARTESIAN_POINT ( 'NONE',  ( -3.458734124999998105, 1.432654583217640276, 19.37500000136560629 ) ) ;
#15344=CARTESIAN_POINT ( 'NONE',  ( 1.656854249492384135, -3.999999999999999112, 11.43750000273119660 ) ) ;
#15348=DIRECTION ( 'NONE',  ( -1.000000000000000000, 0.000000000000000000, 0.000000000000000000 ) ) ;
#15352=CARTESIAN_POINT ( 'NONE',  ( 1.656854249492384135, -3.999999999999999112, 13.31250000000001243 ) ) ;
#15361=FACE_OUTER_BOUND ( 'NONE', #7044, .T. ) ;
#15363=CARTESIAN_POINT ( 'NONE',  ( -2.445694354108818303, -2.445694354108820523, 14.56250000136560452 ) ) ;
#15369=CARTESIAN_POINT ( 'NONE',  ( -2.445694354108819191, 2.445694354108820523, 10.31250000136560629 ) ) ;
#15381=EDGE_CURVE ( 'NONE', #19956, #20461, #20342, .T. ) ;
#15384=CARTESIAN_POINT ( 'NONE',  ( -3.458734124999998993, -1.432654583217642497, 16.75000000136560629 ) ) ;
#15392=CARTESIAN_POINT ( 'NONE',  ( -27.50000000000000711, 7.500000000000001776, -31.01025403784447221 ) ) ;
#15395=CARTESIAN_POINT ( 'NONE',  ( -3.999999999999998224, -1.656854249492383246, 11.18750000273119660 ) ) ;
#15406=CARTESIAN_POINT ( 'NONE',  ( -1.656854249492379250, 4.000000000000000000, 11.81250000000001066 ) ) ;
#15408=CARTESIAN_POINT ( 'NONE',  ( 9.920644283265380691E-16, 4.000000000000000000, 14.75000000000000888 ) ) ;
#15416=CARTESIAN_POINT ( 'NONE',  ( -2.445694354108818303, -2.445694354108820967, 18.81250000136560629 ) ) ;
#15422=CARTESIAN_POINT ( 'NONE',  ( -2.445694354108818303, -2.445694354108820967, 11.81250000136560629 ) ) ;
#15429=CARTESIAN_POINT ( 'NONE',  ( -3.999999999999999112, 0.000000000000000000, 18.12500000273119483 ) ) ;
#15434=CARTESIAN_POINT ( 'NONE',  ( -15.00000000000001066, 10.00000000000000000, -49.99999999999999289 ) ) ;
#15447=CARTESIAN_POINT ( 'NONE',  ( 1.025207404391860050E-15, 3.458734125000000326, 17.18750000136560274 ) ) ;
#15462=ORIENTED_EDGE ( 'NONE', *, *, #16016, .T. ) ;
#15472=DIRECTION ( 'NONE',  ( -1.000000000000000000, 0.000000000000000000, 1.982541115402065110E-16 ) ) ;
#15474=CARTESIAN_POINT ( 'NONE',  ( -1.432654583217639610, -3.458734124999999882, 11.62500000136560452 ) ) ;
#15493=CARTESIAN_POINT ( 'NONE',  ( 3.458734125000001658, 4.235727675282972223E-16, 12.18750000136560629 ) ) ;
#15497=FACE_OUTER_BOUND ( 'NONE', #12882, .T. ) ;
#15507=CARTESIAN_POINT ( 'NONE',  ( -2.828427124746189403, 2.828427124746190291, 10.00000000273119660 ) ) ;
#15518=AXIS2_PLACEMENT_3D ( 'NONE', #12335, #5004, #17815 ) ;
#15537=EDGE_CURVE ( 'NONE', #12610, #13749, #1500, .T. ) ;
#15546=CARTESIAN_POINT ( 'NONE',  ( -3.999999999999998224, -1.656854249492383024, 14.06250000000001066 ) ) ;
#15554=DIRECTION ( 'NONE',  ( 1.000000000000000000, 0.000000000000000000, -1.224646799147353207E-16 ) ) ;
#15567=CARTESIAN_POINT ( 'NONE',  ( 1.971781867644420635E-15, -4.000000000000000000, 12.37500000273119838 ) ) ;
#15581=DIRECTION ( 'NONE',  ( -0.000000000000000000, -0.000000000000000000, -1.000000000000000000 ) ) ;
#15582=ORIENTED_EDGE ( 'NONE', *, *, #19459, .F. ) ;
#15587=DIRECTION ( 'NONE',  ( 0.000000000000000000, 0.000000000000000000, 1.000000000000000000 ) ) ;
#15594=CARTESIAN_POINT ( 'NONE',  ( 3.458734125000001214, 1.432654583217640498, 13.00000000136560452 ) ) ;
#15597=FACE_OUTER_BOUND ( 'NONE', #12126, .T. ) ;
#15599=CARTESIAN_POINT ( 'NONE',  ( -27.50000000000000711, 4.500000000000001776, -33.66025403784446723 ) ) ;
#15601=CARTESIAN_POINT ( 'NONE',  ( -1.432654583217638944, 3.458734125000000326, 10.25000000136560452 ) ) ;
#15603=EDGE_CURVE ( 'NONE', #20532, #11553, #17198, .T. ) ;
#15614=CARTESIAN_POINT ( 'NONE',  ( 3.458734125000001658, 1.432654583217640498, 12.25000000136560452 ) ) ;
#15623=FACE_OUTER_BOUND ( 'NONE', #5079, .T. ) ;
#15627=CARTESIAN_POINT ( 'NONE',  ( 1.656854249492384135, -3.999999999999999112, 12.43750000273119838 ) ) ;
#15636=ORIENTED_EDGE ( 'NONE', *, *, #19475, .T. ) ;
#15639=CARTESIAN_POINT ( 'NONE',  ( -3.999999999999999112, 1.656854249492380582, 19.93750000000001066 ) ) ;
#15646=VECTOR ( 'NONE', #17658, 1000.000000000000000 ) ;
#15648=CARTESIAN_POINT ( 'NONE',  ( 2.445694354108822299, -2.445694354108820079, 19.06250000136560629 ) ) ;
#15649=CARTESIAN_POINT ( 'NONE',  ( 4.000000000000000888, 1.656854249492381248, 15.68750000273119660 ) ) ;
#15663=CARTESIAN_POINT ( 'NONE',  ( 1.656854249492384135, -3.999999999999999112, 15.43750000273119660 ) ) ;
#15665=VERTEX_POINT ( 'NONE', #17722 ) ;
#15670=CARTESIAN_POINT ( 'NONE',  ( -3.999999999999999112, 0.000000000000000000, 18.00000000000001066 ) ) ;
#15673=AXIS2_PLACEMENT_3D ( 'NONE', #13552, #10082, #20819 ) ;
#15675=AXIS2_PLACEMENT_3D ( 'NONE', #1178, #19263, #3098 ) ;
#15684=CARTESIAN_POINT ( 'NONE',  ( -1.432654583217638944, 3.458734125000000326, 19.25000000136560629 ) ) ;
#15688=CARTESIAN_POINT ( 'NONE',  ( 0.9413949561959079615, 0.3373062947069093709, -19.99999999999999645 ) ) ;
#15695=CARTESIAN_POINT ( 'NONE',  ( 4.000000000000001776, -1.656854249492379694, 11.56250000273119660 ) ) ;
#15707=EDGE_CURVE ( 'NONE', #7114, #7929, #1438, .T. ) ;
#15713=CARTESIAN_POINT ( 'NONE',  ( -1.656854249492380138, -3.999999999999999112, 10.31250000273119660 ) ) ;
#15715=CARTESIAN_POINT ( 'NONE',  ( 3.458734125000001214, 1.432654583217640498, 11.00000000136560452 ) ) ;
#15719=AXIS2_PLACEMENT_3D ( 'NONE', #10940, #17869, #3370 ) ;
#15726=CARTESIAN_POINT ( 'NONE',  ( 4.000000000000000888, 4.898587196589412829E-16, 13.62500000273119660 ) ) ;
#15727=ORIENTED_EDGE ( 'NONE', *, *, #12899, .F. ) ;
#15731=CARTESIAN_POINT ( 'NONE',  ( -3.999999999999999112, 0.000000000000000000, 11.00000000000001066 ) ) ;
#15734=CARTESIAN_POINT ( 'NONE',  ( 2.445694354108821411, 2.445694354108820523, 12.31250000136560629 ) ) ;
#15747=CARTESIAN_POINT ( 'NONE',  ( 9.920644283265380691E-16, 4.000000000000000000, 10.87500000273119660 ) ) ;
#15765=CARTESIAN_POINT ( 'NONE',  ( -3.458734124999999437, 1.432654583217640498, 17.62500000136560274 ) ) ;
#15766=CARTESIAN_POINT ( 'NONE',  ( 2.828427124746192067, -2.828427124746189847, 13.50000000273119660 ) ) ;
#15781=ORIENTED_EDGE ( 'NONE', *, *, #12756, .F. ) ;
#15792=CYLINDRICAL_SURFACE ( 'NONE', #8424, 4.000000000000000000 ) ;
#15795=CARTESIAN_POINT ( 'NONE',  ( 1.872352939448454495E-15, -3.458734125000000326, 15.68750000136560629 ) ) ;
#15804=CARTESIAN_POINT ( 'NONE',  ( -2.828427124746189403, 2.828427124746190291, 14.00000000273119660 ) ) ;
#15821=CARTESIAN_POINT ( 'NONE',  ( 3.458734125000001658, 4.235727675282972223E-16, 19.18750000136560629 ) ) ;
#15832=EDGE_LOOP ( 'NONE', ( #19834, #20241, #16214, #21895 ) ) ;
#15836=EDGE_LOOP ( 'NONE', ( #19305, #4269, #5988, #23255 ) ) ;
#15839=EDGE_CURVE ( 'NONE', #15665, #4019, #9945, .T. ) ;
#15841=CARTESIAN_POINT ( 'NONE',  ( -2.445694354108818303, -2.445694354108820967, 12.81250000136560629 ) ) ;
#15846=DIRECTION ( 'NONE',  ( 0.000000000000000000, -0.000000000000000000, -1.000000000000000000 ) ) ;
#15853=CARTESIAN_POINT ( 'NONE',  ( 1.432654583217643163, -3.458734124999999437, 17.75000000136560629 ) ) ;
#15862=CARTESIAN_POINT ( 'NONE',  ( 19.99999999999999289, 4.500000000000003553, -20.00000000000000355 ) ) ;
#15873=CARTESIAN_POINT ( 'NONE',  ( -1.432654583217639166, 3.458734125000000770, 15.50000000136560807 ) ) ;
#15874=CARTESIAN_POINT ( 'NONE',  ( 1.656854249492381470, 4.000000000000000000, 10.81250000273119660 ) ) ;
#15876=DIRECTION ( 'NONE',  ( -0.000000000000000000, 1.000000000000000000, -0.000000000000000000 ) ) ;
#15879=CARTESIAN_POINT ( 'NONE',  ( 1.872352939448454495E-15, -3.458734125000000770, 11.93750000136560629 ) ) ;
#15895=CARTESIAN_POINT ( 'NONE',  ( 4.000000000000001776, -1.656854249492379694, 12.43750000000001066 ) ) ;
#15904=CARTESIAN_POINT ( 'NONE',  ( 1.025207404391860050E-15, 3.458734125000000326, 13.18750000136560452 ) ) ;
#15915=ORIENTED_EDGE ( 'NONE', *, *, #16382, .T. ) ;
#15922=CARTESIAN_POINT ( 'NONE',  ( 2.828427124746192067, -2.828427124746189847, 16.37500000000001066 ) ) ;
#15930=CARTESIAN_POINT ( 'NONE',  ( -3.458734124999998993, 1.432654583217640276, 11.37500000136560452 ) ) ;
#15943=DIRECTION ( 'NONE',  ( -0.000000000000000000, -0.000000000000000000, -1.000000000000000000 ) ) ;
#15945=CARTESIAN_POINT ( 'NONE',  ( 1.432654583217641386, 3.458734125000000770, 13.37500000136560452 ) ) ;
#15961=CARTESIAN_POINT ( 'NONE',  ( -2.445694354108819191, 2.445694354108820523, 17.31250000136560274 ) ) ;
#15964=CARTESIAN_POINT ( 'NONE',  ( 4.000000000000000888, 1.656854249492381248, 16.68750000273119838 ) ) ;
#15974=VERTEX_POINT ( 'NONE', #11615 ) ;
#15983=CARTESIAN_POINT ( 'NONE',  ( 2.445694354108821411, 2.445694354108820523, 15.31250000136560452 ) ) ;
#15984=CARTESIAN_POINT ( 'NONE',  ( -3.999999999999998224, -1.656854249492383246, 10.18750000273119660 ) ) ;
#16002=LINE ( 'NONE', #19927, #11704 ) ;
#16011=CARTESIAN_POINT ( 'NONE',  ( 2.828427124746192067, -2.828427124746189847, 11.37500000000001066 ) ) ;
#16012=ORIENTED_EDGE ( 'NONE', *, *, #21597, .T. ) ;
#16016=EDGE_CURVE ( 'NONE', #14633, #11306, #20313, .T. ) ;
#16022=CARTESIAN_POINT ( 'NONE',  ( 1.025207404391860050E-15, 3.458734125000000326, 14.18750000136560452 ) ) ;
#16025=CYLINDRICAL_SURFACE ( 'NONE', #11728, 4.000000000000000000 ) ;
#16048=LINE ( 'NONE', #6947, #5689 ) ;
#16050=DIRECTION ( 'NONE',  ( -1.000000000000000000, 0.000000000000000000, 1.224646799147353207E-16 ) ) ;
#16051=CARTESIAN_POINT ( 'NONE',  ( 1.432654583217641386, 3.458734125000000770, 19.37500000136560274 ) ) ;
#16070=CARTESIAN_POINT ( 'NONE',  ( 4.000000000000000888, 1.656854249492381248, 17.56250000000001421 ) ) ;
#16073=AXIS2_PLACEMENT_3D ( 'NONE', #3071, #1256, #17580 ) ;
#16077=AXIS2_PLACEMENT_3D ( 'NONE', #18273, #1857, #7516 ) ;
#16085=CARTESIAN_POINT ( 'NONE',  ( -3.458734124999998993, 0.000000000000000000, 18.43750000136560629 ) ) ;
#16108=CARTESIAN_POINT ( 'NONE',  ( 2.445694354108821411, 2.445694354108820523, 16.31250000136560629 ) ) ;
#16109=CARTESIAN_POINT ( 'NONE',  ( -3.999999999999999112, 0.000000000000000000, 11.12500000273119660 ) ) ;
#16118=DIRECTION ( 'NONE',  ( -0.000000000000000000, 1.000000000000000000, -0.000000000000000000 ) ) ;
#16122=( NAMED_UNIT ( * ) SI_UNIT ( $, .STERADIAN. ) SOLID_ANGLE_UNIT ( ) );
#16127=CARTESIAN_POINT ( 'NONE',  ( -3.999999999999999112, 1.656854249492380804, 18.93750000000000711 ) ) ;
#16131=ADVANCED_FACE ( 'NONE', ( #8488 ), #15792, .T. ) ;
#16133=VECTOR ( 'NONE', #14505, 1000.000000000000000 ) ;
#16135=CARTESIAN_POINT ( 'NONE',  ( 9.920644283265380691E-16, 4.000000000000000000, 11.75000000000001066 ) ) ;
#16139=FACE_OUTER_BOUND ( 'NONE', #20141, .T. ) ;
#16143=CARTESIAN_POINT ( 'NONE',  ( 3.458734125000001214, 4.235727675282971730E-16, 13.93750000136560629 ) ) ;
#16153=ADVANCED_FACE ( 'NONE', ( #801 ), #19586, .T. ) ;
#16157=VERTEX_POINT ( 'NONE', #19126 ) ;
#16175=CARTESIAN_POINT ( 'NONE',  ( 4.000000000000000888, 4.898587196589412829E-16, 10.62500000273119660 ) ) ;
#16180=FACE_OUTER_BOUND ( 'NONE', #3310, .T. ) ;
#16184=CARTESIAN_POINT ( 'NONE',  ( -1.656854249492379472, 4.000000000000000000, 12.93750000273119660 ) ) ;
#16185=CARTESIAN_POINT ( 'NONE',  ( 1.656854249492381470, 4.000000000000000000, 19.68750000000001066 ) ) ;
#16196=( BOUNDED_CURVE ( )  B_SPLINE_CURVE ( 2, ( #14023, #9974, #22992, #4670, #2631, #1065, #19383, #10331, #21171 ),
 .UNSPECIFIED., .F., .F. ) 
 B_SPLINE_CURVE_WITH_KNOTS ( ( 3, 2, 2, 2, 3 ),
 ( 0.4000000000000000222, 0.4124999999999999778, 0.4249999999999999889, 0.4375000000000000000, 0.4500000000000000111 ),
 .UNSPECIFIED. ) 
 CURVE ( )  GEOMETRIC_REPRESENTATION_ITEM ( )  RATIONAL_B_SPLINE_CURVE ( ( 1.000000000000000000, 0.9238795325112867385, 1.000000000000000000, 0.9238795325112867385, 1.000000000000000000, 0.9238795325112867385, 1.000000000000000000, 0.9238795325112867385, 1.000000000000000000 ) ) 
 REPRESENTATION_ITEM ( '' )  );
#16199=CARTESIAN_POINT ( 'NONE',  ( -0.9413949561959077394, -0.3373062947069099260, -19.99999999999999645 ) ) ;
#16200=CARTESIAN_POINT ( 'NONE',  ( -3.458734124999998993, 0.000000000000000000, 17.43750000136560274 ) ) ;
#16211=VECTOR ( 'NONE', #2248, 1000.000000000000000 ) ;
#16214=ORIENTED_EDGE ( 'NONE', *, *, #20930, .T. ) ;
#16219=CARTESIAN_POINT ( 'NONE',  ( -1.432654583217639832, -3.458734125000000326, 16.87500000136560629 ) ) ;
#16221=CARTESIAN_POINT ( 'NONE',  ( 4.000000000000001776, -1.656854249492379694, 10.56250000273119660 ) ) ;
#16226=CARTESIAN_POINT ( 'NONE',  ( -3.999999999999999112, 0.000000000000000000, 18.12500000273119483 ) ) ;
#16235=FACE_OUTER_BOUND ( 'NONE', #17768, .T. ) ;
#16237=CARTESIAN_POINT ( 'NONE',  ( -3.999999999999999112, 1.656854249492380804, 16.93750000000001066 ) ) ;
#16242=ORIENTED_EDGE ( 'NONE', *, *, #20190, .T. ) ;
#16244=CARTESIAN_POINT ( 'NONE',  ( 4.000000000000000888, 4.898587196589412829E-16, 12.50000000000001066 ) ) ;
#16258=CARTESIAN_POINT ( 'NONE',  ( -3.458734124999998105, -1.432654583217642275, 14.50000000136560629 ) ) ;
#16282=CARTESIAN_POINT ( 'NONE',  ( -2.828427124746188515, -2.828427124746190735, 18.25000000273119483 ) ) ;
#16307=( BOUNDED_SURFACE ( )  B_SPLINE_SURFACE ( 1, 2, ( 
 ( #13163, #20673, #9574, #5956, #4035, #15197, #11368, #18645, #11501, #9329, #554, #22461, #4278, #11611, #16621, #19810, #1487, #5446, #19929, #16127, #21843, #9298, #18377, #12891, #16585, #22060, #13012, #23648, #1720, #10756, #12781, #7263, #9061, #12673, #23412, #51, #12547, #23526, #3412, #11214, #10863, #21948, #8829, #11093, #14580, #18030, #7137, #1606, #7016, #20276, #8949, #16237, #21716, #14451, #16352, #20034, #5329, #7495, #3529, #3638, #1958, #14332, #164, #18140, #10975, #18251, #1836, #9187, #16473, #14811, #7384, #5677, #3880, #14692, #5561, #20147, #3751, #21595, #5207, #16702, #15285, #22669, #11338, #13597, #9889, #18962, #20863, #4117, #22557, #20513, #4244, #2544, #17183, #764, #4469, #11457, #6165, #18733, #11579, #8095, #6281, #18489, #5920, #2195, #22426, #18846, #2071, #278, #2432, #11691, #9412, #7613, #16830, #22189, #14935, #5803, #9764, #20391, #15167, #17063, #2322, #7736, #13487, #409, #13131, #523, #9655, #3998, #13366, #18608, #4354, #9532, #16945, #15406, #15052, #22308, #13249, #7843, #6039, #20635, #634, #7966, #20749, #7533, #11250, #13056, #1881, #1991, #87, #9447, #14497 ),
 ( #9226, #20312, #22103, #16624, #3913, #2110, #16742, #3677, #5484, #21760, #16509, #11014, #12819, #16394, #19851, #3802, #16282, #3567, #23574, #14978, #14616, #9334, #5245, #14849, #18298, #5371, #10903, #7182, #12589, #323, #12713, #19965, #1764, #18182, #20077, #7420, #9102, #18525, #23692, #14731, #5724, #10793, #7655, #21877, #7308, #21990, #5604, #12930, #20193, #3456, #11140, #18068, #1648, #18414, #202, #8992, #998, #15649, #4038, #20429, #19320, #3035, #15091, #17667, #8330, #22920, #22230, #16871, #10256, #1228, #13851, #5839, #6532, #8566, #21106, #17432, #6648, #12054, #4721, #23037, #1113, #21220, #11371, #13961, #18648, #20552, #2909, #8459, #558, #19210, #9578, #17550, #15766, #13166, #2798, #447, #2237, #7772, #22346, #10382, #5959, #13285, #4158, #4835, #12166, #19437, #11505, #11945, #18776, #2357, #20676, #9689, #16985, #7882, #15200, #22465, #6077, #13409, #4609, #10140, #21825, #23632, #12530, #12651, #10737, #20017, #1347, #5311, #14561, #19911, #16109, #6760, #18123, #5072, #8683, #15874, #10495, #18236, #14076, #16221, #12765, #1819, #3619, #17776, #21700, #15984, #10959, #19556, #23393, #8811, #19792 ) ),
 .UNSPECIFIED., .F., .F., .F. ) 
 B_SPLINE_SURFACE_WITH_KNOTS ( ( 2, 2 ),
 ( 3, 2, 2, 2, 2, 2, 2, 2, 2, 2, 2, 2, 2, 2, 2, 2, 2, 2, 2, 2, 2, 2, 2, 2, 2, 2, 2, 2, 2, 2, 2, 2, 2, 2, 2, 2, 2, 2, 2, 2, 2, 2, 2, 2, 2, 2, 2, 2, 2, 2, 2, 2, 2, 2, 2, 2, 2, 2, 2, 2, 2, 2, 2, 2, 2, 2, 2, 2, 2, 2, 2, 2, 2, 2, 2, 3 ),
 ( 0.000000000000000000, 1.000000000000000000 ),
 ( -0.009250000000000001277, 0.000000000000000000, 0.01250000000000000069, 0.02500000000000000139, 0.03749999999999999861, 0.05000000000000000278, 0.06250000000000000000, 0.07499999999999999722, 0.08749999999999999445, 0.1000000000000000056, 0.1125000000000000028, 0.1250000000000000000, 0.1375000000000000111, 0.1499999999999999944, 0.1625000000000000056, 0.1749999999999999889, 0.1875000000000000000, 0.2000000000000000111, 0.2124999999999999944, 0.2250000000000000056, 0.2374999999999999889, 0.2500000000000000000, 0.2625000000000000111, 0.2750000000000000222, 0.2874999999999999778, 0.2999999999999999889, 0.3125000000000000000, 0.3250000000000000111, 0.3375000000000000222, 0.3499999999999999778, 0.3624999999999999889, 0.3750000000000000000, 0.3875000000000000111, 0.4000000000000000222, 0.4124999999999999778, 0.4249999999999999889, 0.4375000000000000000, 0.4500000000000000111, 0.4625000000000000222, 0.4749999999999999778, 0.4874999999999999889, 0.5000000000000000000, 0.5124999999999999556, 0.5250000000000000222, 0.5374999999999999778, 0.5500000000000000444, 0.5625000000000000000, 0.5749999999999999556, 0.5875000000000000222, 0.5999999999999999778, 0.6125000000000000444, 0.6250000000000000000, 0.6374999999999999556, 0.6500000000000000222, 0.6624999999999999778, 0.6750000000000000444, 0.6875000000000000000, 0.6999999999999999556, 0.7125000000000000222, 0.7249999999999999778, 0.7375000000000000444, 0.7500000000000000000, 0.7624999999999999556, 0.7750000000000000222, 0.7874999999999999778, 0.8000000000000000444, 0.8125000000000000000, 0.8249999999999999556, 0.8375000000000000222, 0.8499999999999999778, 0.8625000000000000444, 0.8750000000000000000, 0.8874999999999999556, 0.9000000000000000222, 0.9124999999999999778, 0.9250000000000000444 ),
 .UNSPECIFIED. ) 
 GEOMETRIC_REPRESENTATION_ITEM ( )  RATIONAL_B_SPLINE_SURFACE ( (
 ( 1.000000000000000000, 1.000000000000000000, 1.000000000000000000, 0.9238795325112867385, 1.000000000000000000, 0.9238795325112867385, 1.000000000000000000, 0.9238795325112867385, 1.000000000000000000, 0.9238795325112867385, 1.000000000000000000, 0.9238795325112867385, 1.000000000000000000, 0.9238795325112867385, 1.000000000000000000, 0.9238795325112867385, 1.000000000000000000, 0.9238795325112867385, 1.000000000000000000, 0.9238795325112867385, 1.000000000000000000, 0.9238795325112867385, 1.000000000000000000, 0.9238795325112867385, 1.000000000000000000, 0.9238795325112867385, 1.000000000000000000, 0.9238795325112867385, 1.000000000000000000, 0.9238795325112867385, 1.000000000000000000, 0.9238795325112867385, 1.000000000000000000, 0.9238795325112867385, 1.000000000000000000, 0.9238795325112867385, 1.000000000000000000, 0.9238795325112867385, 1.000000000000000000, 0.9238795325112867385, 1.000000000000000000, 0.9238795325112867385, 1.000000000000000000, 0.9238795325112867385, 1.000000000000000000, 0.9238795325112867385, 1.000000000000000000, 0.9238795325112867385, 1.000000000000000000, 0.9238795325112867385, 1.000000000000000000, 0.9238795325112867385, 1.000000000000000000, 0.9238795325112867385, 1.000000000000000000, 0.9238795325112867385, 1.000000000000000000, 0.9238795325112867385, 1.000000000000000000, 0.9238795325112867385, 1.000000000000000000, 0.9238795325112867385, 1.000000000000000000, 0.9238795325112867385, 1.000000000000000000, 0.9238795325112867385, 1.000000000000000000, 0.9238795325112867385, 1.000000000000000000, 0.9238795325112867385, 1.000000000000000000, 0.9238795325112867385, 1.000000000000000000, 0.9238795325112867385, 1.000000000000000000, 0.9238795325112867385, 1.000000000000000000, 0.9238795325112867385, 1.000000000000000000, 0.9238795325112867385, 1.000000000000000000, 0.9238795325112867385, 1.000000000000000000, 0.9238795325112867385, 1.000000000000000000, 0.9238795325112867385, 1.000000000000000000, 0.9238795325112867385, 1.000000000000000000, 0.9238795325112867385, 1.000000000000000000, 0.9238795325112867385, 1.000000000000000000, 0.9238795325112867385, 1.000000000000000000, 0.9238795325112867385, 1.000000000000000000, 0.9238795325112867385, 1.000000000000000000, 0.9238795325112867385, 1.000000000000000000, 0.9238795325112867385, 1.000000000000000000, 0.9238795325112867385, 1.000000000000000000, 0.9238795325112867385, 1.000000000000000000, 0.9238795325112867385, 1.000000000000000000, 0.9238795325112867385, 1.000000000000000000, 0.9238795325112867385, 1.000000000000000000, 0.9238795325112867385, 1.000000000000000000, 0.9238795325112867385, 1.000000000000000000, 0.9238795325112867385, 1.000000000000000000, 0.9238795325112867385, 1.000000000000000000, 0.9238795325112867385, 1.000000000000000000, 0.9238795325112867385, 1.000000000000000000, 0.9238795325112867385, 1.000000000000000000, 0.9238795325112867385, 1.000000000000000000, 0.9238795325112867385, 1.000000000000000000, 0.9238795325112867385, 1.000000000000000000, 0.9238795325112867385, 1.000000000000000000, 0.9238795325112867385, 1.000000000000000000, 0.9238795325112867385, 1.000000000000000000, 0.9238795325112867385, 1.000000000000000000, 0.9238795325112867385, 1.000000000000000000, 0.9238795325112867385, 1.000000000000000000, 0.9238795325112867385, 1.000000000000000000, 0.9238795325112867385, 1.000000000000000000, 0.9238795325112867385, 1.000000000000000000),
 ( 1.000000000000000000, 1.000000000000000000, 1.000000000000000000, 0.9238795325112867385, 1.000000000000000000, 0.9238795325112867385, 1.000000000000000000, 0.9238795325112867385, 1.000000000000000000, 0.9238795325112867385, 1.000000000000000000, 0.9238795325112867385, 1.000000000000000000, 0.9238795325112867385, 1.000000000000000000, 0.9238795325112867385, 1.000000000000000000, 0.9238795325112867385, 1.000000000000000000, 0.9238795325112867385, 1.000000000000000000, 0.9238795325112867385, 1.000000000000000000, 0.9238795325112867385, 1.000000000000000000, 0.9238795325112867385, 1.000000000000000000, 0.9238795325112867385, 1.000000000000000000, 0.9238795325112867385, 1.000000000000000000, 0.9238795325112867385, 1.000000000000000000, 0.9238795325112867385, 1.000000000000000000, 0.9238795325112867385, 1.000000000000000000, 0.9238795325112867385, 1.000000000000000000, 0.9238795325112867385, 1.000000000000000000, 0.9238795325112867385, 1.000000000000000000, 0.9238795325112867385, 1.000000000000000000, 0.9238795325112867385, 1.000000000000000000, 0.9238795325112867385, 1.000000000000000000, 0.9238795325112867385, 1.000000000000000000, 0.9238795325112867385, 1.000000000000000000, 0.9238795325112867385, 1.000000000000000000, 0.9238795325112867385, 1.000000000000000000, 0.9238795325112867385, 1.000000000000000000, 0.9238795325112867385, 1.000000000000000000, 0.9238795325112867385, 1.000000000000000000, 0.9238795325112867385, 1.000000000000000000, 0.9238795325112867385, 1.000000000000000000, 0.9238795325112867385, 1.000000000000000000, 0.9238795325112867385, 1.000000000000000000, 0.9238795325112867385, 1.000000000000000000, 0.9238795325112867385, 1.000000000000000000, 0.9238795325112867385, 1.000000000000000000, 0.9238795325112867385, 1.000000000000000000, 0.9238795325112867385, 1.000000000000000000, 0.9238795325112867385, 1.000000000000000000, 0.9238795325112867385, 1.000000000000000000, 0.9238795325112867385, 1.000000000000000000, 0.9238795325112867385, 1.000000000000000000, 0.9238795325112867385, 1.000000000000000000, 0.9238795325112867385, 1.000000000000000000, 0.9238795325112867385, 1.000000000000000000, 0.9238795325112867385, 1.000000000000000000, 0.9238795325112867385, 1.000000000000000000, 0.9238795325112867385, 1.000000000000000000, 0.9238795325112867385, 1.000000000000000000, 0.9238795325112867385, 1.000000000000000000, 0.9238795325112867385, 1.000000000000000000, 0.9238795325112867385, 1.000000000000000000, 0.9238795325112867385, 1.000000000000000000, 0.9238795325112867385, 1.000000000000000000, 0.9238795325112867385, 1.000000000000000000, 0.9238795325112867385, 1.000000000000000000, 0.9238795325112867385, 1.000000000000000000, 0.9238795325112867385, 1.000000000000000000, 0.9238795325112867385, 1.000000000000000000, 0.9238795325112867385, 1.000000000000000000, 0.9238795325112867385, 1.000000000000000000, 0.9238795325112867385, 1.000000000000000000, 0.9238795325112867385, 1.000000000000000000, 0.9238795325112867385, 1.000000000000000000, 0.9238795325112867385, 1.000000000000000000, 0.9238795325112867385, 1.000000000000000000, 0.9238795325112867385, 1.000000000000000000, 0.9238795325112867385, 1.000000000000000000, 0.9238795325112867385, 1.000000000000000000, 0.9238795325112867385, 1.000000000000000000, 0.9238795325112867385, 1.000000000000000000, 0.9238795325112867385, 1.000000000000000000, 0.9238795325112867385, 1.000000000000000000) ) ) 
 REPRESENTATION_ITEM ( '' )  SURFACE ( )  );
#16308=CARTESIAN_POINT ( 'NONE',  ( 4.000000000000000888, 4.898587196589412829E-16, 19.50000000000001066 ) ) ;
#16315=CARTESIAN_POINT ( 'NONE',  ( 1.432654583217643163, -3.458734124999999437, 16.75000000136560629 ) ) ;
#16320=CARTESIAN_POINT ( 'NONE',  ( 2.445694354108821411, 2.445694354108820523, 16.06250000136560629 ) ) ;
#16335=CARTESIAN_POINT ( 'NONE',  ( -2.445694354108819191, 2.445694354108820523, 13.56250000136560629 ) ) ;
#16340=CARTESIAN_POINT ( 'NONE',  ( -3.999999999999999112, 1.656854249492380804, 19.06250000273119483 ) ) ;
#16352=CARTESIAN_POINT ( 'NONE',  ( 9.920644283265380691E-16, 4.000000000000000000, 16.75000000000001066 ) ) ;
#16366=DIRECTION ( 'NONE',  ( 1.224646799147353207E-16, 0.000000000000000000, 1.000000000000000000 ) ) ;
#16377=ORIENTED_EDGE ( 'NONE', *, *, #20093, .F. ) ;
#16380=ADVANCED_FACE ( 'NONE', ( #17921 ), #23425, .F. ) ;
#16382=EDGE_CURVE ( 'NONE', #14730, #14629, #10646, .T. ) ;
#16394=CARTESIAN_POINT ( 'NONE',  ( 1.656854249492384135, -3.999999999999999112, 18.43750000273119483 ) ) ;
#16396=DIRECTION ( 'NONE',  ( 1.000000000000000000, 0.000000000000000000, 0.000000000000000000 ) ) ;
#16415=CARTESIAN_POINT ( 'NONE',  ( 4.000000000000000888, 4.898587196589412829E-16, 19.50000000000001066 ) ) ;
#16418=AXIS2_PLACEMENT_3D ( 'NONE', #12580, #14487, #14721 ) ;
#16419=CARTESIAN_POINT ( 'NONE',  ( 1.025207404391860050E-15, 3.458734125000000770, 10.43750000136560629 ) ) ;
#16428=CARTESIAN_POINT ( 'NONE',  ( -3.458734124999998993, 0.000000000000000000, 19.43750000136560629 ) ) ;
#16430=MECHANICAL_DESIGN_GEOMETRIC_PRESENTATION_REPRESENTATION('',(#1876),#20235);
#16434=CARTESIAN_POINT ( 'NONE',  ( 1.432654583217643163, -3.458734124999999437, 14.75000000136560452 ) ) ;
#16438=VERTEX_POINT ( 'NONE', #20403 ) ;
#16443=AXIS2_PLACEMENT_3D ( 'NONE', #13662, #1280, #8271 ) ;
#16455=CARTESIAN_POINT ( 'NONE',  ( -2.445694354108819191, 2.445694354108820523, 11.56250000136560629 ) ) ;
#16461=CARTESIAN_POINT ( 'NONE',  ( 1.971781867644420635E-15, -4.000000000000000000, 17.37500000273119483 ) ) ;
#16469=AXIS2_PLACEMENT_3D ( 'NONE', #2776, #977, #4700 ) ;
#16471=CARTESIAN_POINT ( 'NONE',  ( 9.920644283265380691E-16, 4.000000000000000000, 9.875000002731196602 ) ) ;
#16473=CARTESIAN_POINT ( 'NONE',  ( -2.828427124746189403, 2.828427124746190291, 15.87500000000001066 ) ) ;
#16488=CARTESIAN_POINT ( 'NONE',  ( 1.872352939448454495E-15, -3.458734125000000326, 10.68750000136560452 ) ) ;
#16490=CARTESIAN_POINT ( 'NONE',  ( 2.828427124746192067, -2.828427124746189847, 18.50000000273119483 ) ) ;
#16506=PLANE ( 'NONE',  #11814 ) ;
#16509=CARTESIAN_POINT ( 'NONE',  ( 4.000000000000000888, 4.898587196589412829E-16, 18.62500000273119483 ) ) ;
#16515=DIRECTION ( 'NONE',  ( 1.224646799147353207E-16, -0.000000000000000000, 1.000000000000000000 ) ) ;
#16520=LINE ( 'NONE', #10911, #9703 ) ;
#16525=VERTEX_POINT ( 'NONE', #2332 ) ;
#16532=CARTESIAN_POINT ( 'NONE',  ( 19.99999999999998934, 9.999999999999964473, -50.00000000000000000 ) ) ;
#16533=CARTESIAN_POINT ( 'NONE',  ( 2.828427124746191179, 2.828427124746190291, 17.62500000000001066 ) ) ;
#16545=CARTESIAN_POINT ( 'NONE',  ( -1.432654583217638944, 3.458734125000000326, 16.25000000136560629 ) ) ;
#16549=CARTESIAN_POINT ( 'NONE',  ( 3.458734125000002102, -1.432654583217639610, 12.87500000136560629 ) ) ;
#16561=CARTESIAN_POINT ( 'NONE',  ( 3.458734125000001658, 1.432654583217640498, 19.25000000136560274 ) ) ;
#16565=CARTESIAN_POINT ( 'NONE',  ( 3.458734125000001658, 4.235727675282972223E-16, 13.18750000136560452 ) ) ;
#16571=( BOUNDED_CURVE ( )  B_SPLINE_CURVE ( 2, ( #20212, #16888, #20691, #2484, #4295, #18429, #5975, #16637, #11632 ),
 .UNSPECIFIED., .F., .F. ) 
 B_SPLINE_CURVE_WITH_KNOTS ( ( 3, 2, 2, 2, 3 ),
 ( 0.4000000000000000222, 0.4124999999999999778, 0.4249999999999999889, 0.4375000000000000000, 0.4500000000000000111 ),
 .UNSPECIFIED. ) 
 CURVE ( )  GEOMETRIC_REPRESENTATION_ITEM ( )  RATIONAL_B_SPLINE_CURVE ( ( 1.000000000000000000, 0.9238795325112867385, 1.000000000000000000, 0.9238795325112867385, 1.000000000000000000, 0.9238795325112867385, 1.000000000000000000, 0.9238795325112867385, 1.000000000000000000 ) ) 
 REPRESENTATION_ITEM ( '' )  );
#16573=CARTESIAN_POINT ( 'NONE',  ( 1.656854249492384135, -3.999999999999999112, 17.43750000273119483 ) ) ;
#16585=CARTESIAN_POINT ( 'NONE',  ( 2.828427124746191179, 2.828427124746190291, 18.62500000000001066 ) ) ;
#16587=AXIS2_PLACEMENT_3D ( 'NONE', #23105, #7076, #12609 ) ;
#16590=( NAMED_UNIT ( * ) PLANE_ANGLE_UNIT ( ) SI_UNIT ( $, .RADIAN. ) );
#16592=CARTESIAN_POINT ( 'NONE',  ( -35.00000000000000000, 4.500000000000001776, -19.99999999999998934 ) ) ;
#16600=CARTESIAN_POINT ( 'NONE',  ( -2.445694354108819191, 2.445694354108820523, 13.56250000136560629 ) ) ;
#16604=CARTESIAN_POINT ( 'NONE',  ( -3.999999999999999112, 1.656854249492380582, 16.93750000000001066 ) ) ;
#16605=ORIENTED_EDGE ( 'NONE', *, *, #19420, .F. ) ;
#16614=EDGE_LOOP ( 'NONE', ( #22336, #19785, #8252, #13884 ) ) ;
#16621=CARTESIAN_POINT ( 'NONE',  ( 1.971781867644420635E-15, -4.000000000000000000, 19.25000000000001066 ) ) ;
#16624=CARTESIAN_POINT ( 'NONE',  ( -3.999999999999999112, 1.656854249492380804, 19.06250000273119483 ) ) ;
#16637=CARTESIAN_POINT ( 'NONE',  ( 4.000000000000000888, 1.656854249492381248, 14.68750000273119660 ) ) ;
#16647=CARTESIAN_POINT ( 'NONE',  ( 2.828427124746192067, -2.828427124746189847, 16.37500000000001066 ) ) ;
#16649=FACE_OUTER_BOUND ( 'NONE', #4595, .T. ) ;
#16659=CARTESIAN_POINT ( 'NONE',  ( 2.445694354108821855, -2.445694354108820079, 15.81250000136560629 ) ) ;
#16663=CARTESIAN_POINT ( 'NONE',  ( -27.50000000000000711, 7.500000000000002665, -31.01025403784447576 ) ) ;
#16664=CARTESIAN_POINT ( 'NONE',  ( -3.458734124999998993, 0.000000000000000000, 14.43750000136560452 ) ) ;
#16680=CARTESIAN_POINT ( 'NONE',  ( 2.445694354108822299, -2.445694354108820079, 16.06250000136560629 ) ) ;
#16684=ADVANCED_FACE ( 'NONE', ( #8218 ), #13854, .F. ) ;
#16686=CARTESIAN_POINT ( 'NONE',  ( -2.445694354108819191, 2.445694354108820523, 10.56250000136560629 ) ) ;
#16689=CARTESIAN_POINT ( 'NONE',  ( -20.00000000000001066, 9.999999999999964473, -49.99999999999999289 ) ) ;
#16690=CARTESIAN_POINT ( 'NONE',  ( 1.432654583217643163, -3.458734124999999437, 11.75000000136560629 ) ) ;
#16691=CARTESIAN_POINT ( 'NONE',  ( 4.000000000000000888, 1.656854249492381248, 17.68750000273119483 ) ) ;
#16702=CARTESIAN_POINT ( 'NONE',  ( -1.656854249492380138, -3.999999999999999112, 15.18750000000001066 ) ) ;
#16716=CARTESIAN_POINT ( 'NONE',  ( 1.025207404391860050E-15, 3.458734125000000770, 13.43750000136560452 ) ) ;
#16722=CARTESIAN_POINT ( 'NONE',  ( -1.656854249492379472, 4.000000000000000000, 11.93750000273119660 ) ) ;
#16724=LINE ( 'NONE', #303, #19629 ) ;
#16742=CARTESIAN_POINT ( 'NONE',  ( 9.920644283265380691E-16, 4.000000000000000000, 18.87500000273119838 ) ) ;
#16749=CARTESIAN_POINT ( 'NONE',  ( -2.762848947613220307, 4.746226468750993632, -26.84672628368516811 ) ) ;
#16762=CARTESIAN_POINT ( 'NONE',  ( 1.971781867644420635E-15, -4.000000000000000000, 16.37500000273119838 ) ) ;
#16768=CARTESIAN_POINT ( 'NONE',  ( -1.656854249492380138, -3.999999999999999112, 14.18750000000001066 ) ) ;
#16769=CARTESIAN_POINT ( 'NONE',  ( -3.999999999999999112, 0.000000000000000000, 21.31370849898476649 ) ) ;
#16778=DIRECTION ( 'NONE',  ( -1.000000000000000000, 0.000000000000000000, 0.000000000000000000 ) ) ;
#16780=CARTESIAN_POINT ( 'NONE',  ( -1.432654583217638944, 3.458734125000000326, 17.25000000136560274 ) ) ;
#16785=CARTESIAN_POINT ( 'NONE',  ( 2.828427124746191179, 2.828427124746190291, 12.62500000000001066 ) ) ;
#16786=CARTESIAN_POINT ( 'NONE',  ( 2.445694354108821411, 2.445694354108820523, 13.06250000136560452 ) ) ;
#16800=CARTESIAN_POINT ( 'NONE',  ( 1.025207404391860050E-15, 3.458734125000000770, 15.43750000136560452 ) ) ;
#16809=CARTESIAN_POINT ( 'NONE',  ( 2.445694354108821411, 2.445694354108820523, 13.31250000136560452 ) ) ;
#16817=CARTESIAN_POINT ( 'NONE',  ( 2.828427124746191179, 2.828427124746190291, 17.75000000273119483 ) ) ;
#16827=EDGE_CURVE ( 'NONE', #315, #9317, #7095, .T. ) ;
#16830=CARTESIAN_POINT ( 'NONE',  ( -2.828427124746188515, -2.828427124746190735, 13.12500000000001243 ) ) ;
#16846=CARTESIAN_POINT ( 'NONE',  ( 2.445694354108822299, -2.445694354108820079, 14.06250000136560629 ) ) ;
#16851=CARTESIAN_POINT ( 'NONE',  ( 9.920644283265380691E-16, 4.000000000000000000, 11.87500000273119660 ) ) ;
#16861=ORIENTED_EDGE ( 'NONE', *, *, #7773, .F. ) ;
#16871=CARTESIAN_POINT ( 'NONE',  ( -3.999999999999999112, 1.656854249492380804, 15.06250000273119483 ) ) ;
#16888=CARTESIAN_POINT ( 'NONE',  ( -3.999999999999999112, 1.656854249492380582, 15.06250000273119660 ) ) ;
#16896=CARTESIAN_POINT ( 'NONE',  ( 9.920644283265380691E-16, 4.000000000000000000, 14.75000000000000888 ) ) ;
#16905=CARTESIAN_POINT ( 'NONE',  ( 3.458734125000002102, -1.432654583217639610, 11.87500000136560452 ) ) ;
#16911=CARTESIAN_POINT ( 'NONE',  ( 1.025207404391860050E-15, 3.458734125000000326, 13.18750000136560452 ) ) ;
#16922=VERTEX_POINT ( 'NONE', #12626 ) ;
#16923=CARTESIAN_POINT ( 'NONE',  ( 2.445694354108822299, -2.445694354108820079, 15.06250000136560452 ) ) ;
#16934=CARTESIAN_POINT ( 'NONE',  ( 3.458734125000001214, 1.432654583217640498, 11.00000000136560452 ) ) ;
#16935=CARTESIAN_POINT ( 'NONE',  ( 4.000000000000000888, 4.898587196589412829E-16, 14.62500000273119660 ) ) ;
#16936=CARTESIAN_POINT ( 'NONE',  ( 35.00000000000000000, 4.500000000000001776, -20.00000000000000355 ) ) ;
#16944=ORIENTED_EDGE ( 'NONE', *, *, #14235, .F. ) ;
#16945=CARTESIAN_POINT ( 'NONE',  ( -2.828427124746189403, 2.828427124746190291, 11.87500000000001066 ) ) ;
#16947=CARTESIAN_POINT ( 'NONE',  ( -2.828427124746189403, 2.828427124746190291, 14.87500000000000888 ) ) ;
#16959=CARTESIAN_POINT ( 'NONE',  ( 2.445694354108822299, -2.445694354108820079, 16.06250000136560629 ) ) ;
#16964=CARTESIAN_POINT ( 'NONE',  ( -1.656854249492380138, -3.999999999999999112, 14.18750000000001066 ) ) ;
#16984=ORIENTED_EDGE ( 'NONE', *, *, #23128, .F. ) ;
#16985=CARTESIAN_POINT ( 'NONE',  ( -2.828427124746188515, -2.828427124746190735, 12.25000000273119838 ) ) ;
#16999=LINE ( 'NONE', #20446, #21982 ) ;
#17004=DIRECTION ( 'NONE',  ( -0.000000000000000000, 1.000000000000000000, -0.000000000000000000 ) ) ;
#17008=CARTESIAN_POINT ( 'NONE',  ( -1.656854249492379250, 4.000000000000000000, 12.81250000000001066 ) ) ;
#17018=CARTESIAN_POINT ( 'NONE',  ( 3.458734125000001214, 4.235727675282971730E-16, 14.93750000136560452 ) ) ;
#17026=LINE ( 'NONE', #9976, #9993 ) ;
#17027=ORIENTED_EDGE ( 'NONE', *, *, #20202, .T. ) ;
#17028=CARTESIAN_POINT ( 'NONE',  ( 9.920644283265380691E-16, 4.000000000000000000, 15.87500000273119660 ) ) ;
#17037=CARTESIAN_POINT ( 'NONE',  ( -2.445694354108819191, 2.445694354108820523, 15.56250000136560629 ) ) ;
#17039=ORIENTED_EDGE ( 'NONE', *, *, #3363, .T. ) ;
#17051=CARTESIAN_POINT ( 'NONE',  ( 1.971781867644420635E-15, -4.000000000000000000, 13.37500000273119660 ) ) ;
#17054=CARTESIAN_POINT ( 'NONE',  ( -3.999999999999999112, 0.000000000000000000, 14.00000000000001066 ) ) ;
#17057=CIRCLE ( 'NONE', #6726, 2.649999999999992806 ) ;
#17063=CARTESIAN_POINT ( 'NONE',  ( 1.656854249492381470, 4.000000000000000000, 12.68750000000001243 ) ) ;
#17064=CARTESIAN_POINT ( 'NONE',  ( -3.999999999999999112, 0.000000000000000000, 15.00000000000001066 ) ) ;
#17068=( BOUNDED_CURVE ( )  B_SPLINE_CURVE ( 2, ( #17054, #10239, #17530, #6033, #4462, #11684, #13359, #17297, #10009 ),
 .UNSPECIFIED., .F., .F. ) 
 B_SPLINE_CURVE_WITH_KNOTS ( ( 3, 2, 2, 2, 3 ),
 ( 0.5999999999999999778, 0.6125000000000000444, 0.6250000000000000000, 0.6374999999999999556, 0.6500000000000000222 ),
 .UNSPECIFIED. ) 
 CURVE ( )  GEOMETRIC_REPRESENTATION_ITEM ( )  RATIONAL_B_SPLINE_CURVE ( ( 1.000000000000000000, 0.9238795325112867385, 1.000000000000000000, 0.9238795325112867385, 1.000000000000000000, 0.9238795325112867385, 1.000000000000000000, 0.9238795325112867385, 1.000000000000000000 ) ) 
 REPRESENTATION_ITEM ( '' )  );
#17077=CARTESIAN_POINT ( 'NONE',  ( -2.445694354108819191, 2.445694354108820523, 14.56250000136560452 ) ) ;
#17078=PLANE ( 'NONE',  #17210 ) ;
#17120=CARTESIAN_POINT ( 'NONE',  ( 1.236993788156008760E-15, 0.000000000000000000, 21.31370849898476649 ) ) ;
#17123=CARTESIAN_POINT ( 'NONE',  ( 2.828427124746192067, -2.828427124746189847, 13.37500000000001243 ) ) ;
#17127=CARTESIAN_POINT ( 'NONE',  ( -20.00000000000000711, -10.00000000000000000, -19.99999999999999645 ) ) ;
#17134=LINE ( 'NONE', #9966, #22118 ) ;
#17136=CARTESIAN_POINT ( 'NONE',  ( 1.872352939448454495E-15, -3.458734125000000326, 12.68750000136560629 ) ) ;
#17141=EDGE_CURVE ( 'NONE', #3286, #20917, #18809, .T. ) ;
#17143=CARTESIAN_POINT ( 'NONE',  ( -3.458734124999998993, 0.000000000000000000, 10.43750000136560452 ) ) ;
#17154=ORIENTED_EDGE ( 'NONE', *, *, #9186, .F. ) ;
#17157=ORIENTED_EDGE ( 'NONE', *, *, #16827, .F. ) ;
#17158=CARTESIAN_POINT ( 'NONE',  ( 3.458734125000002546, -1.432654583217639610, 18.12500000136560274 ) ) ;
#17170=CARTESIAN_POINT ( 'NONE',  ( 2.445694354108821855, -2.445694354108820079, 11.81250000136560629 ) ) ;
#17171=CARTESIAN_POINT ( 'NONE',  ( -2.828427124746189403, 2.828427124746190291, 13.00000000273119660 ) ) ;
#17183=CARTESIAN_POINT ( 'NONE',  ( 2.828427124746192067, -2.828427124746189847, 14.37500000000001066 ) ) ;
#17185=VECTOR ( 'NONE', #3326, 1000.000000000000000 ) ;
#17187=CARTESIAN_POINT ( 'NONE',  ( 1.656854249492381470, 4.000000000000000000, 14.68750000000000888 ) ) ;
#17188=ORIENTED_EDGE ( 'NONE', *, *, #9524, .T. ) ;
#17196=CARTESIAN_POINT ( 'NONE',  ( -2.828427124746188515, -2.828427124746190735, 11.12500000000001066 ) ) ;
#17198=CIRCLE ( 'NONE', #15675, 4.999999999999999112 ) ;
#17202=CARTESIAN_POINT ( 'NONE',  ( -3.458734124999999437, 1.432654583217640498, 10.62500000136560452 ) ) ;
#17210=AXIS2_PLACEMENT_3D ( 'NONE', #9550, #9311, #652 ) ;
#17216=( BOUNDED_CURVE ( )  B_SPLINE_CURVE ( 2, ( #1012, #22935, #17563, #15663, #1127, #19335, #21236, #6549, #4848 ),
 .UNSPECIFIED., .F., .F. ) 
 B_SPLINE_CURVE_WITH_KNOTS ( ( 3, 2, 2, 2, 3 ),
 ( 0.3499999999999999778, 0.3624999999999999889, 0.3750000000000000000, 0.3875000000000000111, 0.4000000000000000222 ),
 .UNSPECIFIED. ) 
 CURVE ( )  GEOMETRIC_REPRESENTATION_ITEM ( )  RATIONAL_B_SPLINE_CURVE ( ( 1.000000000000000000, 0.9238795325112867385, 1.000000000000000000, 0.9238795325112867385, 1.000000000000000000, 0.9238795325112867385, 1.000000000000000000, 0.9238795325112867385, 1.000000000000000000 ) ) 
 REPRESENTATION_ITEM ( '' )  );
#17225=VECTOR ( 'NONE', #14209, 1000.000000000000000 ) ;
#17227=VERTEX_POINT ( 'NONE', #17493 ) ;
#17237=CARTESIAN_POINT ( 'NONE',  ( -3.999999999999998224, -1.656854249492383024, 12.06250000000001066 ) ) ;
#17249=CARTESIAN_POINT ( 'NONE',  ( 2.828427124746191179, 2.828427124746190291, 11.62500000000001066 ) ) ;
#17259=CARTESIAN_POINT ( 'NONE',  ( 1.971781867644420635E-15, -4.000000000000000000, 10.37500000273119660 ) ) ;
#17262=CARTESIAN_POINT ( 'NONE',  ( 3.458734125000001214, 1.432654583217640498, 12.00000000136560452 ) ) ;
#17280=CARTESIAN_POINT ( 'NONE',  ( -3.458734124999999437, 0.000000000000000000, 14.68750000136560452 ) ) ;
#17281=CARTESIAN_POINT ( 'NONE',  ( 4.000000000000000888, 4.898587196589412829E-16, 12.62500000273119660 ) ) ;
#17294=CARTESIAN_POINT ( 'NONE',  ( 9.920644283265380691E-16, 4.000000000000000000, 13.87500000273119483 ) ) ;
#17297=CARTESIAN_POINT ( 'NONE',  ( 4.000000000000000888, 1.656854249492381248, 13.56250000000001066 ) ) ;
#17303=VERTEX_POINT ( 'NONE', #19507 ) ;
#17312=CARTESIAN_POINT ( 'NONE',  ( -2.828427124746188515, -2.828427124746190735, 15.12500000000001066 ) ) ;
#17315=CARTESIAN_POINT ( 'NONE',  ( 2.828427124746192067, -2.828427124746189847, 11.37500000000001066 ) ) ;
#17326=DIRECTION ( 'NONE',  ( 1.000000000000000000, 0.000000000000000000, -1.224646799147353207E-16 ) ) ;
#17329=FILL_AREA_STYLE ('',( #11957 ) ) ;
#17333=PLANE ( 'NONE',  #9110 ) ;
#17345=CARTESIAN_POINT ( 'NONE',  ( -1.656854249492380138, -3.999999999999999112, 12.31250000273120015 ) ) ;
#17346=CARTESIAN_POINT ( 'NONE',  ( -3.458734124999998105, -1.432654583217642275, 17.50000000136560274 ) ) ;
#17350=CARTESIAN_POINT ( 'NONE',  ( -3.999999999999999112, 0.000000000000000000, 21.31370849898476649 ) ) ;
#17351=( BOUNDED_CURVE ( )  B_SPLINE_CURVE ( 2, ( #20587, #19033, #4428, #4664, #17259, #15713, #9838, #19264, #10202 ),
 .UNSPECIFIED., .F., .F. ) 
 B_SPLINE_CURVE_WITH_KNOTS ( ( 3, 2, 2, 2, 3 ),
 ( 0.8499999999999999778, 0.8625000000000000444, 0.8750000000000000000, 0.8874999999999999556, 0.9000000000000000222 ),
 .UNSPECIFIED. ) 
 CURVE ( )  GEOMETRIC_REPRESENTATION_ITEM ( )  RATIONAL_B_SPLINE_CURVE ( ( 1.000000000000000000, 0.9238795325112867385, 1.000000000000000000, 0.9238795325112867385, 1.000000000000000000, 0.9238795325112867385, 1.000000000000000000, 0.9238795325112867385, 1.000000000000000000 ) ) 
 REPRESENTATION_ITEM ( '' )  );
#17370=CARTESIAN_POINT ( 'NONE',  ( 35.00000000000000000, 7.500000000000001776, -20.00000000000000355 ) ) ;
#17372=CARTESIAN_POINT ( 'NONE',  ( 1.025207404391860050E-15, 3.458734125000000326, 15.18750000136560452 ) ) ;
#17375=CARTESIAN_POINT ( 'NONE',  ( 14.99999999999999289, 10.00000000000000000, -50.00000000000000000 ) ) ;
#17381=PRODUCT_DEFINITION_SHAPE ( 'NONE', 'NONE',  #20705 ) ;
#17384=DIRECTION ( 'NONE',  ( 1.224646799147353207E-16, -0.000000000000000000, 1.000000000000000000 ) ) ;
#17392=CARTESIAN_POINT ( 'NONE',  ( -1.432654583217639832, -3.458734125000000326, 11.87500000136560452 ) ) ;
#17407=CARTESIAN_POINT ( 'NONE',  ( -3.999999999999999112, 1.656854249492380804, 13.06250000273119660 ) ) ;
#17409=ORIENTED_EDGE ( 'NONE', *, *, #9390, .F. ) ;
#17418=ORIENTED_EDGE ( 'NONE', *, *, #18855, .T. ) ;
#17431=CARTESIAN_POINT ( 'NONE',  ( -1.432654583217639166, 3.458734125000000770, 18.50000000136560629 ) ) ;
#17432=CARTESIAN_POINT ( 'NONE',  ( 4.000000000000001776, -1.656854249492379694, 14.56250000273119660 ) ) ;
#17446=VERTEX_POINT ( 'NONE', #21995 ) ;
#17448=SURFACE_STYLE_USAGE ( .BOTH. , #10155 ) ;
#17463=ORIENTED_EDGE ( 'NONE', *, *, #20093, .T. ) ;
#17478=DIRECTION ( 'NONE',  ( -1.000000000000000000, 0.000000000000000000, 0.000000000000000000 ) ) ;
#17480=DIRECTION ( 'NONE',  ( -1.224646799147353207E-16, 0.000000000000000000, -1.000000000000000000 ) ) ;
#17488=VERTEX_POINT ( 'NONE', #207 ) ;
#17492=CARTESIAN_POINT ( 'NONE',  ( 3.458734125000002546, -1.432654583217639610, 17.12500000136560629 ) ) ;
#17493=CARTESIAN_POINT ( 'NONE',  ( -0.3649867057748643617, 3.983313282257324950, 10.00000000000000888 ) ) ;
#17506=ORIENTED_EDGE ( 'NONE', *, *, #14362, .F. ) ;
#17511=CARTESIAN_POINT ( 'NONE',  ( -2.445694354108819191, 2.445694354108820523, 12.56250000136560629 ) ) ;
#17515=PLANE ( 'NONE',  #4137 ) ;
#17516=EDGE_CURVE ( 'NONE', #17488, #19299, #4400, .T. ) ;
#17523=CARTESIAN_POINT ( 'NONE',  ( 4.000000000000001776, -1.656854249492379694, 13.43750000000001243 ) ) ;
#17525=CARTESIAN_POINT ( 'NONE',  ( -1.656854249492379250, 4.000000000000000000, 13.93750000273119483 ) ) ;
#17530=CARTESIAN_POINT ( 'NONE',  ( -2.828427124746189403, 2.828427124746190291, 13.87500000000001066 ) ) ;
#17548=CARTESIAN_POINT ( 'NONE',  ( 3.458734125000002546, -1.432654583217639610, 18.12500000136560274 ) ) ;
#17550=CARTESIAN_POINT ( 'NONE',  ( 4.000000000000001776, -1.656854249492379694, 13.56250000273119660 ) ) ;
#17563=CARTESIAN_POINT ( 'NONE',  ( 2.828427124746192067, -2.828427124746189847, 15.50000000273119660 ) ) ;
#17580=DIRECTION ( 'NONE',  ( 1.000000000000000000, 0.000000000000000000, 0.000000000000000000 ) ) ;
#17581=CIRCLE ( 'NONE', #20986, 4.999999999999999112 ) ;
#17585=CARTESIAN_POINT ( 'NONE',  ( 1.025207404391860050E-15, 3.458734125000000326, 16.18750000136560629 ) ) ;
#17599=VERTEX_POINT ( 'NONE', #3918 ) ;
#17601=VERTEX_POINT ( 'NONE', #2117 ) ;
#17602=CARTESIAN_POINT ( 'NONE',  ( -1.656854249492379472, 4.000000000000000000, 17.81250000000001066 ) ) ;
#17605=CARTESIAN_POINT ( 'NONE',  ( 2.828427124746192067, -2.828427124746189847, 19.37500000000001066 ) ) ;
#17615=CARTESIAN_POINT ( 'NONE',  ( 2.445694354108821411, 2.445694354108820523, 11.06250000136560452 ) ) ;
#17621=AXIS2_PLACEMENT_3D ( 'NONE', #18569, #2152, #11417 ) ;
#17628=CARTESIAN_POINT ( 'NONE',  ( -2.828427124746188515, -2.828427124746190735, 13.25000000273119660 ) ) ;
#17629=ORIENTED_EDGE ( 'NONE', *, *, #3302, .T. ) ;
#17635=CARTESIAN_POINT ( 'NONE',  ( 3.458734125000001658, 1.432654583217640498, 11.25000000136560452 ) ) ;
#17648=CARTESIAN_POINT ( 'NONE',  ( -3.458734124999998993, 1.432654583217640276, 19.37500000136560274 ) ) ;
#17658=DIRECTION ( 'NONE',  ( 1.000000000000000000, -0.000000000000000000, -1.224646799147353207E-16 ) ) ;
#17660=CARTESIAN_POINT ( 'NONE',  ( -2.828427124746189403, 2.828427124746190291, 19.87500000000001066 ) ) ;
#17666=CARTESIAN_POINT ( 'NONE',  ( 1.432654583217643163, -3.458734124999999882, 15.00000000136560807 ) ) ;
#17667=CARTESIAN_POINT ( 'NONE',  ( -1.656854249492380138, -3.999999999999999112, 15.31250000273119660 ) ) ;
#17672=CARTESIAN_POINT ( 'NONE',  ( -1.432654583217639832, -3.458734125000000326, 11.87500000136560452 ) ) ;
#17674=VERTEX_POINT ( 'NONE', #2363 ) ;
#17686=DIRECTION ( 'NONE',  ( 0.000000000000000000, 0.000000000000000000, 1.000000000000000000 ) ) ;
#17698=CARTESIAN_POINT ( 'NONE',  ( -2.445694354108819191, 2.445694354108820523, 15.31250000136560452 ) ) ;
#17713=ORIENTED_EDGE ( 'NONE', *, *, #18855, .F. ) ;
#17722=CARTESIAN_POINT ( 'NONE',  ( 4.000000000000000888, 4.898587196589412829E-16, -20.00000000000000000 ) ) ;
#17725=CARTESIAN_POINT ( 'NONE',  ( -1.432654583217638944, 3.458734125000000326, 11.25000000136560452 ) ) ;
#17728=VERTEX_POINT ( 'NONE', #19590 ) ;
#17730=VECTOR ( 'NONE', #149, 1000.000000000000000 ) ;
#17739=ORIENTED_EDGE ( 'NONE', *, *, #15839, .F. ) ;
#17743=CARTESIAN_POINT ( 'NONE',  ( 1.025207404391860050E-15, 3.458734125000000770, 11.43750000136560452 ) ) ;
#17747=DIRECTION ( 'NONE',  ( -1.000000000000000000, 0.000000000000000000, 0.000000000000000000 ) ) ;
#17755=CARTESIAN_POINT ( 'NONE',  ( 1.872352939448454495E-15, -3.458734125000000326, 15.68750000136560629 ) ) ;
#17758=CARTESIAN_POINT ( 'NONE',  ( -3.999999999999998224, -1.656854249492383024, 14.18750000273119660 ) ) ;
#17768=EDGE_LOOP ( 'NONE', ( #8575, #1782, #3317, #7040 ) ) ;
#17775=CARTESIAN_POINT ( 'NONE',  ( 1.872352939448454495E-15, -3.458734125000000770, 14.93750000136560452 ) ) ;
#17776=CARTESIAN_POINT ( 'NONE',  ( -1.656854249492380138, -3.999999999999999112, 10.31250000273119483 ) ) ;
#17787=ORIENTED_EDGE ( 'NONE', *, *, #8357, .F. ) ;
#17797=ORIENTED_EDGE ( 'NONE', *, *, #14235, .T. ) ;
#17798=DIRECTION ( 'NONE',  ( -0.000000000000000000, -0.000000000000000000, -1.000000000000000000 ) ) ;
#17799=CARTESIAN_POINT ( 'NONE',  ( 4.000000000000000888, 1.656854249492381248, 11.56250000000001066 ) ) ;
#17809=CARTESIAN_POINT ( 'NONE',  ( 3.458734125000002102, -1.432654583217639610, 12.87500000136560629 ) ) ;
#17815=DIRECTION ( 'NONE',  ( 1.000000000000000000, 0.000000000000000000, 0.000000000000000000 ) ) ;
#17834=DIRECTION ( 'NONE',  ( 1.000000000000000000, -0.000000000000000000, -1.224646799147353207E-16 ) ) ;
#17836=CARTESIAN_POINT ( 'NONE',  ( 1.432654583217643163, -3.458734124999999882, 18.00000000136560274 ) ) ;
#17839=ORIENTED_EDGE ( 'NONE', *, *, #5962, .F. ) ;
#17843=DIRECTION ( 'NONE',  ( 1.000000000000000000, 0.000000000000000000, 0.000000000000000000 ) ) ;
#17852=CARTESIAN_POINT ( 'NONE',  ( 4.000000000000000888, 1.656854249492381248, 12.68750000273119660 ) ) ;
#17854=CARTESIAN_POINT ( 'NONE',  ( -3.999999999999999112, 0.000000000000000000, 18.00000000000001066 ) ) ;
#17868=CARTESIAN_POINT ( 'NONE',  ( -3.458734124999998993, -1.432654583217642497, 17.50000000136560274 ) ) ;
#17869=DIRECTION ( 'NONE',  ( -0.000000000000000000, 1.000000000000000000, -0.000000000000000000 ) ) ;
#17886=CARTESIAN_POINT ( 'NONE',  ( -3.999999999999999112, 0.000000000000000000, 14.12500000273119660 ) ) ;
#17889=CARTESIAN_POINT ( 'NONE',  ( -1.432654583217639166, 3.458734125000000770, 17.50000000136560274 ) ) ;
#17902=CARTESIAN_POINT ( 'NONE',  ( 1.025207404391860050E-15, 3.458734125000000326, 10.18750000136560629 ) ) ;
#17905=CARTESIAN_POINT ( 'NONE',  ( -35.00000000000000711, 4.500000000000001776, -49.99999999999998579 ) ) ;
#17910=DIRECTION ( 'NONE',  ( 0.8660254037844385966, 0.000000000000000000, 0.5000000000000001110 ) ) ;
#17913=CYLINDRICAL_SURFACE ( 'NONE', #1491, 4.000000000000000000 ) ;
#17915=AXIS2_PLACEMENT_3D ( 'NONE', #23256, #6866, #988 ) ;
#17916=CARTESIAN_POINT ( 'NONE',  ( -2.828427124746188515, -2.828427124746190735, 12.12500000000001066 ) ) ;
#17921=FACE_OUTER_BOUND ( 'NONE', #19172, .T. ) ;
#17925=CARTESIAN_POINT ( 'NONE',  ( 3.458734125000001214, 4.235727675282971730E-16, 14.93750000136560452 ) ) ;
#17935=ORIENTED_EDGE ( 'NONE', *, *, #8210, .F. ) ;
#17938=EDGE_LOOP ( 'NONE', ( #2062, #23259, #5736, #4737 ) ) ;
#17954=CARTESIAN_POINT ( 'NONE',  ( 1.025207404391860050E-15, 3.458734125000000326, 10.18750000136560629 ) ) ;
#17958=ORIENTED_EDGE ( 'NONE', *, *, #10708, .F. ) ;
#17961=CARTESIAN_POINT ( 'NONE',  ( 4.000000000000000888, 1.656854249492381248, 10.68750000273119483 ) ) ;
#17970=EDGE_CURVE ( 'NONE', #4949, #12476, #673, .T. ) ;
#17974=CARTESIAN_POINT ( 'NONE',  ( 2.828427124746192067, -2.828427124746189847, 18.37500000000001066 ) ) ;
#17977=AXIS2_PLACEMENT_3D ( 'NONE', #3303, #18152, #16366 ) ;
#17980=CARTESIAN_POINT ( 'NONE',  ( 34.99999999999999289, 7.500000000000001776, -50.00000000000000000 ) ) ;
#17990=CARTESIAN_POINT ( 'NONE',  ( -1.432654583217639610, -3.458734124999999882, 16.62500000136560629 ) ) ;
#18004=ORIENTED_EDGE ( 'NONE', *, *, #396, .T. ) ;
#18012=( BOUNDED_CURVE ( )  B_SPLINE_CURVE ( 2, ( #645, #6050, #17315, #9902, #15061, #20649, #17196, #2442, #8107 ),
 .UNSPECIFIED., .F., .F. ) 
 B_SPLINE_CURVE_WITH_KNOTS ( ( 3, 2, 2, 2, 3 ),
 ( 0.8499999999999999778, 0.8625000000000000444, 0.8750000000000000000, 0.8874999999999999556, 0.9000000000000000222 ),
 .UNSPECIFIED. ) 
 CURVE ( )  GEOMETRIC_REPRESENTATION_ITEM ( )  RATIONAL_B_SPLINE_CURVE ( ( 1.000000000000000000, 0.9238795325112867385, 1.000000000000000000, 0.9238795325112867385, 1.000000000000000000, 0.9238795325112867385, 1.000000000000000000, 0.9238795325112867385, 1.000000000000000000 ) ) 
 REPRESENTATION_ITEM ( '' )  );
#18013=CARTESIAN_POINT ( 'NONE',  ( 3.458734125000001658, 1.432654583217640498, 17.25000000136560629 ) ) ;
#18019=CARTESIAN_POINT ( 'NONE',  ( -3.999999999999998224, -1.656854249492383246, 18.18750000273119483 ) ) ;
#18030=CARTESIAN_POINT ( 'NONE',  ( 1.656854249492384135, -3.999999999999999112, 17.31250000000001421 ) ) ;
#18034=ORIENTED_EDGE ( 'NONE', *, *, #8764, .T. ) ;
#18036=CARTESIAN_POINT ( 'NONE',  ( -3.999999999999999112, 1.656854249492380804, 11.93750000000001066 ) ) ;
#18047=CARTESIAN_POINT ( 'NONE',  ( -1.432654583217639610, -3.458734124999999882, 13.62500000136560452 ) ) ;
#18066=CARTESIAN_POINT ( 'NONE',  ( -3.999999999999999112, 0.000000000000000000, 12.12500000273119838 ) ) ;
#18068=CARTESIAN_POINT ( 'NONE',  ( -3.999999999999999112, 1.656854249492380804, 16.06250000273119838 ) ) ;
#18071=CARTESIAN_POINT ( 'NONE',  ( 35.00000000000000000, 7.500000000000001776, -20.00000000000000355 ) ) ;
#18087=LINE ( 'NONE', #1784, #4892 ) ;
#18088=CARTESIAN_POINT ( 'NONE',  ( 4.000000000000000888, 1.656854249492381248, 18.56250000000001421 ) ) ;
#18103=CARTESIAN_POINT ( 'NONE',  ( -1.432654583217638944, 3.458734125000000326, 16.25000000136560629 ) ) ;
#18111=( BOUNDED_CURVE ( )  B_SPLINE_CURVE ( 2, ( #14522, #1551, #7082, #14399, #21662, #21786, #5393, #3477, #12733 ),
 .UNSPECIFIED., .F., .F. ) 
 B_SPLINE_CURVE_WITH_KNOTS ( ( 3, 2, 2, 2, 3 ),
 ( 0.1000000000000000056, 0.1125000000000000028, 0.1250000000000000000, 0.1375000000000000111, 0.1499999999999999944 ),
 .UNSPECIFIED. ) 
 CURVE ( )  GEOMETRIC_REPRESENTATION_ITEM ( )  RATIONAL_B_SPLINE_CURVE ( ( 1.000000000000000000, 0.9238795325112867385, 1.000000000000000000, 0.9238795325112867385, 1.000000000000000000, 0.9238795325112867385, 1.000000000000000000, 0.9238795325112867385, 1.000000000000000000 ) ) 
 REPRESENTATION_ITEM ( '' )  );
#18122=CARTESIAN_POINT ( 'NONE',  ( 1.432654583217641386, 3.458734125000000770, 14.37500000136560452 ) ) ;
#18123=CARTESIAN_POINT ( 'NONE',  ( -2.828427124746189403, 2.828427124746190291, 11.00000000273119660 ) ) ;
#18125=DIRECTION ( 'NONE',  ( 0.000000000000000000, 0.000000000000000000, 1.000000000000000000 ) ) ;
#18129=CARTESIAN_POINT ( 'NONE',  ( 2.828427124746191179, 2.828427124746190291, 18.75000000273119483 ) ) ;
#18132=CARTESIAN_POINT ( 'NONE',  ( -3.999999999999999112, 0.000000000000000000, 16.00000000000001066 ) ) ;
#18139=ORIENTED_EDGE ( 'NONE', *, *, #21361, .T. ) ;
#18140=CARTESIAN_POINT ( 'NONE',  ( -1.656854249492380138, -3.999999999999999112, 16.18750000000001066 ) ) ;
#18142=CARTESIAN_POINT ( 'NONE',  ( -3.729367062499998831, 0.000000000000000000, 19.28125000204840234 ) ) ;
#18144=ORIENTED_EDGE ( 'NONE', *, *, #10920, .F. ) ;
#18152=DIRECTION ( 'NONE',  ( -1.000000000000000000, 0.000000000000000000, 1.224646799147353207E-16 ) ) ;
#18158=CARTESIAN_POINT ( 'NONE',  ( 1.432654583217643163, -3.458734124999999437, 10.75000000136560452 ) ) ;
#18162=CARTESIAN_POINT ( 'NONE',  ( -3.999999999999999112, 1.656854249492380582, 12.06250000273119838 ) ) ;
#18172=CARTESIAN_POINT ( 'NONE',  ( 2.828427124746192067, -2.828427124746189847, 18.37500000000001066 ) ) ;
#18182=CARTESIAN_POINT ( 'NONE',  ( -3.999999999999998224, -1.656854249492383246, 17.18750000273119838 ) ) ;
#18191=CARTESIAN_POINT ( 'NONE',  ( 1.236993788156008760E-15, 0.000000000000000000, 21.31370849898476649 ) ) ;
#18201=ORIENTED_EDGE ( 'NONE', *, *, #12899, .T. ) ;
#18202=CYLINDRICAL_SURFACE ( 'NONE', #11064, 2.649999999999992806 ) ;
#18203=EDGE_LOOP ( 'NONE', ( #5498, #8915 ) ) ;
#18207=CARTESIAN_POINT ( 'NONE',  ( 1.656854249492381470, 4.000000000000000000, 18.68750000000001066 ) ) ;
#18208=CARTESIAN_POINT ( 'NONE',  ( 19.99999999999999289, 9.999999999999964473, -20.00000000000000355 ) ) ;
#18214=CARTESIAN_POINT ( 'NONE',  ( -3.458734124999998993, 0.000000000000000000, 16.43750000136560629 ) ) ;
#18217=CARTESIAN_POINT ( 'NONE',  ( -1.665216334060555692, 3.652639802690383242, 9.999838423880746063 ) ) ;
#18218=CARTESIAN_POINT ( 'NONE',  ( 1.025207404391860050E-15, 3.458734125000000326, 12.18750000136560629 ) ) ;
#18226=CARTESIAN_POINT ( 'NONE',  ( 4.000000000000000888, 4.898587196589412829E-16, 17.50000000000001066 ) ) ;
#18236=CARTESIAN_POINT ( 'NONE',  ( 4.000000000000000888, 1.656854249492381248, 10.68750000273119483 ) ) ;
#18247=( NAMED_UNIT ( * ) PLANE_ANGLE_UNIT ( ) SI_UNIT ( $, .RADIAN. ) );
#18251=CARTESIAN_POINT ( 'NONE',  ( -3.999999999999998224, -1.656854249492383246, 16.06250000000001066 ) ) ;
#18255=( LENGTH_UNIT ( ) NAMED_UNIT ( * ) SI_UNIT ( .MILLI., .METRE. ) );
#18256=VECTOR ( 'NONE', #19431, 1000.000000000000000 ) ;
#18273=CARTESIAN_POINT ( 'NONE',  ( 0.000000000000000000, 0.000000000000000000, 20.00000000000001066 ) ) ;
#18277=VECTOR ( 'NONE', #11340, 1000.000000000000000 ) ;
#18283=VERTEX_POINT ( 'NONE', #12208 ) ;
#18285=ORIENTED_EDGE ( 'NONE', *, *, #19407, .T. ) ;
#18292=AXIS2_PLACEMENT_3D ( 'NONE', #6730, #12024, #17747 ) ;
#18298=CARTESIAN_POINT ( 'NONE',  ( 2.828427124746191179, 2.828427124746190291, 17.75000000273119483 ) ) ;
#18318=VERTEX_POINT ( 'NONE', #20906 ) ;
#18324=CARTESIAN_POINT ( 'NONE',  ( 2.828427124746191179, 2.828427124746190291, 18.62500000000001066 ) ) ;
#18328=CIRCLE ( 'NONE', #14528, 2.649999999999989253 ) ;
#18336=CARTESIAN_POINT ( 'NONE',  ( 1.025207404391860050E-15, 3.458734125000000326, 18.18750000136560274 ) ) ;
#18339=MECHANICAL_DESIGN_GEOMETRIC_PRESENTATION_REPRESENTATION('',(#8032),#6848);
#18342=CARTESIAN_POINT ( 'NONE',  ( 1.872352939448454495E-15, -3.458734125000000326, 14.68750000136560452 ) ) ;
#18344=ORIENTED_EDGE ( 'NONE', *, *, #11430, .T. ) ;
#18351=CARTESIAN_POINT ( 'NONE',  ( 4.000000000000001776, -1.656854249492379694, 17.43750000000001066 ) ) ;
#18354=CARTESIAN_POINT ( 'NONE',  ( -3.999999999999999112, 0.000000000000000000, 15.00000000000001066 ) ) ;
#18360=CARTESIAN_POINT ( 'NONE',  ( 3.458734125000002546, -1.432654583217639610, 13.12500000136560629 ) ) ;
#18366=CARTESIAN_POINT ( 'NONE',  ( 9.920644283265380691E-16, 4.000000000000000000, 16.87500000273119838 ) ) ;
#18369=ORIENTED_EDGE ( 'NONE', *, *, #13492, .T. ) ;
#18377=CARTESIAN_POINT ( 'NONE',  ( 9.920644283265380691E-16, 4.000000000000000000, 18.75000000000001066 ) ) ;
#18386=DIRECTION ( 'NONE',  ( -1.000000000000000000, 0.000000000000000000, 0.000000000000000000 ) ) ;
#18390=CARTESIAN_POINT ( 'NONE',  ( -3.458734124999998993, -1.432654583217642497, 13.75000000136560452 ) ) ;
#18414=CARTESIAN_POINT ( 'NONE',  ( -1.656854249492379250, 4.000000000000000000, 15.93750000273119838 ) ) ;
#18429=CARTESIAN_POINT ( 'NONE',  ( 1.656854249492381470, 4.000000000000000000, 14.81250000273119838 ) ) ;
#18434=CARTESIAN_POINT ( 'NONE',  ( 14.99999999999995559, -15.00000000000000000, -50.00000000000000000 ) ) ;
#18437=LINE ( 'NONE', #16532, #20573 ) ;
#18438=CARTESIAN_POINT ( 'NONE',  ( 1.656854249492384135, -3.999999999999999112, 16.31250000000001066 ) ) ;
#18441=CARTESIAN_POINT ( 'NONE',  ( 1.656854249492381470, 4.000000000000000000, 17.81250000273119483 ) ) ;
#18448=CARTESIAN_POINT ( 'NONE',  ( -3.458734124999998993, 1.432654583217640276, 16.37500000136560629 ) ) ;
#18455=CARTESIAN_POINT ( 'NONE',  ( 1.432654583217641164, 3.458734125000000326, 13.12500000136560274 ) ) ;
#18464=CARTESIAN_POINT ( 'NONE',  ( 1.971781867644420635E-15, -4.000000000000000000, 17.25000000000001066 ) ) ;
#18472=CARTESIAN_POINT ( 'NONE',  ( 3.458734125000001658, 4.235727675282972223E-16, 12.18750000136560629 ) ) ;
#18477=CARTESIAN_POINT ( 'NONE',  ( 1.971781867644420635E-15, -4.000000000000000000, 16.37500000273119838 ) ) ;
#18485=VECTOR ( 'NONE', #1318, 1000.000000000000000 ) ;
#18489=CARTESIAN_POINT ( 'NONE',  ( -1.656854249492379250, 4.000000000000000000, 13.81250000000001066 ) ) ;
#18501=CARTESIAN_POINT ( 'NONE',  ( 3.458734125000002546, -1.432654583217639610, 14.12500000136560452 ) ) ;
#18525=CARTESIAN_POINT ( 'NONE',  ( -1.656854249492379250, 4.000000000000000000, 16.93750000273119838 ) ) ;
#18535=CARTESIAN_POINT ( 'NONE',  ( 4.000000000000001776, -1.656854249492379694, 12.43750000000001066 ) ) ;
#18543=VECTOR ( 'NONE', #20590, 1000.000000000000000 ) ;
#18544=CARTESIAN_POINT ( 'NONE',  ( -1.656854249492380138, -3.999999999999999112, 16.31250000273119838 ) ) ;
#18549=CARTESIAN_POINT ( 'NONE',  ( 9.920644283265380691E-16, 4.000000000000000000, 15.75000000000001066 ) ) ;
#18551=ADVANCED_FACE ( 'NONE', ( #14116 ), #16025, .T. ) ;
#18560=FACE_OUTER_BOUND ( 'NONE', #10179, .T. ) ;
#18563=CARTESIAN_POINT ( 'NONE',  ( -3.458734124999998993, -1.432654583217642497, 15.50000000136560807 ) ) ;
#18568=CARTESIAN_POINT ( 'NONE',  ( -2.445694354108819191, 2.445694354108820523, 14.31250000136560452 ) ) ;
#18569=CARTESIAN_POINT ( 'NONE',  ( 1.236993788156008760E-15, 0.000000000000000000, 21.31370849898476649 ) ) ;
#18572=VERTEX_POINT ( 'NONE', #7400 ) ;
#18583=VECTOR ( 'NONE', #9553, 1000.000000000000000 ) ;
#18584=CARTESIAN_POINT ( 'NONE',  ( 1.432654583217641386, 3.458734125000000770, 17.37500000136560274 ) ) ;
#18591=CARTESIAN_POINT ( 'NONE',  ( 3.458734125000002546, -1.432654583217639610, 12.12500000136560629 ) ) ;
#18597=CARTESIAN_POINT ( 'NONE',  ( 3.458734125000001214, 4.235727675282971730E-16, 10.93750000136560452 ) ) ;
#18598=CARTESIAN_POINT ( 'NONE',  ( 9.920644283265380691E-16, 4.000000000000000000, 14.87500000273119660 ) ) ;
#18608=CARTESIAN_POINT ( 'NONE',  ( -3.999999999999998224, -1.656854249492383246, 12.06250000000001243 ) ) ;
#18612=CARTESIAN_POINT ( 'NONE',  ( -20.00000000000001066, -10.00000000000000000, -49.99999999999999289 ) ) ;
#18616=EDGE_CURVE ( 'NONE', #2705, #7575, #2359, .T. ) ;
#18623=CARTESIAN_POINT ( 'NONE',  ( 2.445694354108822299, -2.445694354108820079, 13.06250000136560629 ) ) ;
#18645=CARTESIAN_POINT ( 'NONE',  ( 1.656854249492381470, 4.000000000000000000, 19.68750000000001066 ) ) ;
#18647=ORIENTED_EDGE ( 'NONE', *, *, #15707, .T. ) ;
#18648=CARTESIAN_POINT ( 'NONE',  ( -2.828427124746189403, 2.828427124746190291, 14.00000000273119660 ) ) ;
#18661=LINE ( 'NONE', #21887, #16211 ) ;
#18666=CARTESIAN_POINT ( 'NONE',  ( 4.000000000000000888, 4.898587196589412829E-16, 21.31370849898476649 ) ) ;
#18674=CARTESIAN_POINT ( 'NONE',  ( 2.828427124746191179, 2.828427124746190291, 15.62500000000001066 ) ) ;
#18686=CARTESIAN_POINT ( 'NONE',  ( 3.458734125000002102, -1.432654583217639610, 16.87500000136560629 ) ) ;
#18691=CARTESIAN_POINT ( 'NONE',  ( 3.458734125000001214, 4.235727675282971730E-16, 14.93750000136560452 ) ) ;
#18696=ORIENTED_EDGE ( 'NONE', *, *, #20202, .F. ) ;
#18705=CARTESIAN_POINT ( 'NONE',  ( -2.445694354108818303, -2.445694354108820967, 17.81250000136560274 ) ) ;
#18719=CARTESIAN_POINT ( 'NONE',  ( 1.025207404391860050E-15, 3.458734125000000326, 12.18750000136560629 ) ) ;
#18720=CARTESIAN_POINT ( 'NONE',  ( 4.000000000000001776, -1.656854249492379694, 17.56250000273119838 ) ) ;
#18730=EDGE_CURVE ( 'NONE', #14904, #18283, #2213, .T. ) ;
#18733=CARTESIAN_POINT ( 'NONE',  ( -3.999999999999998224, -1.656854249492383246, 14.06250000000001066 ) ) ;
#18735=VECTOR ( 'NONE', #14681, 1000.000000000000000 ) ;
#18737=ORIENTED_EDGE ( 'NONE', *, *, #8357, .T. ) ;
#18752=CARTESIAN_POINT ( 'NONE',  ( 1.432654583217641386, 3.458734125000000770, 15.37500000136560807 ) ) ;
#18773=CARTESIAN_POINT ( 'NONE',  ( -3.999999999999999112, 0.000000000000000000, 17.12500000273119838 ) ) ;
#18775=EDGE_LOOP ( 'NONE', ( #15582, #16984 ) ) ;
#18776=CARTESIAN_POINT ( 'NONE',  ( 2.828427124746192067, -2.828427124746189847, 12.50000000273119838 ) ) ;
#18777=( BOUNDED_SURFACE ( )  B_SPLINE_SURFACE ( 1, 2, ( 
 ( #16428, #7343, #5405, #14767, #121, #11, #14650, #5878, #10935, #1795, #11050, #15011, #20468, #13202, #12742, #7695, #22020, #5636, #3709, #9481, #18336, #9142, #20347, #12969, #9022, #21799, #12849, #3841, #7567, #20231, #19993, #14533, #2146, #23605, #11176, #16780, #361, #3954, #22266, #4074, #11409, #18686, #11288, #16315, #7219, #3595, #7451, #9259, #18214, #18448, #2028, #16545, #20106, #21907, #14887, #5515, #1918, #9368, #16659, #234, #5763, #22144, #13091, #18563, #7806, #4313, #4550, #5994, #17372, #4431, #4196, #22506, #17018, #2506, #8048, #11538, #6357, #6116, #15363, #2744, #15122, #940, #11651, #13446, #11766, #20708, #10084, #482, #8163, #2391, #13554, #19035, #9723, #8279, #9840, #18808, #20821, #13321, #22384, #22744, #6476, #594, #21054, #15594, #22862, #4666, #18917, #13671, #17136, #2624, #9615, #13797, #12000, #15239, #7919, #6233, #9968, #2275, #20589, #17262, #19157, #16905, #712, #22630, #830, #15474, #20934, #11886, #21166, #15930, #10445, #17725, #10325, #2973, #17615, #15715, #1288, #8626, #1181, #8518, #16488, #4778, #12115, #21278, #1534, #7396, #64, #22987, #17954 ),
 ( #6704, #13908, #21965, #19377, #23207, #16051, #14141, #14708, #15821, #6819, #23093, #21406, #19505, #10204, #21524, #14018, #5024, #4902, #12238, #1060, #12354, #19616, #23340, #3103, #8745, #3214, #10561, #17836, #5135, #6949, #1404, #14264, #12472, #19735, #3336, #8398, #10679, #8876, #5577, #19266, #2854, #17492, #6592, #5815, #2210, #20655, #20406, #22321, #5937, #12905, #7511, #536, #15304, #4134, #20165, #13263, #7984, #3891, #16959, #20526, #20290, #11476, #13386, #15182, #11594, #1970, #4259, #9310, #11227, #18752, #22441, #14952, #9549, #180, #2336, #7859, #22578, #423, #5695, #9669, #3772, #11112, #17077, #651, #14824, #22077, #13030, #13142, #2447, #18501, #16846, #6054, #9782, #11351, #18862, #18390, #7750, #9427, #16600, #2087, #16716, #294, #7630, #22204, #4014, #15066, #18623, #1006, #10391, #8113, #11951, #19101, #20997, #6418, #20767, #8467, #2693, #22686, #6182, #780, #8572, #4370, #6541, #3042, #15879, #17672, #15422, #12061, #6298, #1233, #9907, #13733, #22804, #2806, #8222, #11709, #19216, #4617, #13502, #13615, #4729, #23043, #18976, #20877, #8338, #17202, #2559, #2916, #4486 ) ),
 .UNSPECIFIED., .F., .F., .F. ) 
 B_SPLINE_SURFACE_WITH_KNOTS ( ( 2, 2 ),
 ( 3, 2, 2, 2, 2, 2, 2, 2, 2, 2, 2, 2, 2, 2, 2, 2, 2, 2, 2, 2, 2, 2, 2, 2, 2, 2, 2, 2, 2, 2, 2, 2, 2, 2, 2, 2, 2, 2, 2, 2, 2, 2, 2, 2, 2, 2, 2, 2, 2, 2, 2, 2, 2, 2, 2, 2, 2, 2, 2, 2, 2, 2, 2, 2, 2, 2, 2, 2, 2, 2, 2, 2, 2, 2, 3 ),
 ( 0.000000000000000000, 1.000000000000000000 ),
 ( 0.000000000000000000, 0.01250000000000000069, 0.02500000000000000139, 0.03749999999999999861, 0.05000000000000000278, 0.06250000000000000000, 0.07499999999999999722, 0.08749999999999999445, 0.1000000000000000056, 0.1125000000000000028, 0.1250000000000000000, 0.1375000000000000111, 0.1499999999999999944, 0.1625000000000000056, 0.1749999999999999889, 0.1875000000000000000, 0.2000000000000000111, 0.2124999999999999944, 0.2250000000000000056, 0.2374999999999999889, 0.2500000000000000000, 0.2625000000000000111, 0.2750000000000000222, 0.2874999999999999778, 0.2999999999999999889, 0.3125000000000000000, 0.3250000000000000111, 0.3375000000000000222, 0.3499999999999999778, 0.3624999999999999889, 0.3750000000000000000, 0.3875000000000000111, 0.4000000000000000222, 0.4124999999999999778, 0.4249999999999999889, 0.4375000000000000000, 0.4500000000000000111, 0.4625000000000000222, 0.4749999999999999778, 0.4874999999999999889, 0.5000000000000000000, 0.5124999999999999556, 0.5250000000000000222, 0.5374999999999999778, 0.5500000000000000444, 0.5625000000000000000, 0.5749999999999999556, 0.5875000000000000222, 0.5999999999999999778, 0.6125000000000000444, 0.6250000000000000000, 0.6374999999999999556, 0.6500000000000000222, 0.6624999999999999778, 0.6750000000000000444, 0.6875000000000000000, 0.6999999999999999556, 0.7125000000000000222, 0.7249999999999999778, 0.7375000000000000444, 0.7500000000000000000, 0.7624999999999999556, 0.7750000000000000222, 0.7874999999999999778, 0.8000000000000000444, 0.8125000000000000000, 0.8249999999999999556, 0.8375000000000000222, 0.8499999999999999778, 0.8625000000000000444, 0.8750000000000000000, 0.8874999999999999556, 0.9000000000000000222, 0.9124999999999999778, 0.9250000000000000444 ),
 .UNSPECIFIED. ) 
 GEOMETRIC_REPRESENTATION_ITEM ( )  RATIONAL_B_SPLINE_SURFACE ( (
 ( 1.000000000000000000, 0.9238795325112867385, 1.000000000000000000, 0.9238795325112867385, 1.000000000000000000, 0.9238795325112867385, 1.000000000000000000, 0.9238795325112867385, 1.000000000000000000, 0.9238795325112867385, 1.000000000000000000, 0.9238795325112867385, 1.000000000000000000, 0.9238795325112867385, 1.000000000000000000, 0.9238795325112867385, 1.000000000000000000, 0.9238795325112867385, 1.000000000000000000, 0.9238795325112867385, 1.000000000000000000, 0.9238795325112867385, 1.000000000000000000, 0.9238795325112867385, 1.000000000000000000, 0.9238795325112867385, 1.000000000000000000, 0.9238795325112867385, 1.000000000000000000, 0.9238795325112867385, 1.000000000000000000, 0.9238795325112867385, 1.000000000000000000, 0.9238795325112867385, 1.000000000000000000, 0.9238795325112867385, 1.000000000000000000, 0.9238795325112867385, 1.000000000000000000, 0.9238795325112867385, 1.000000000000000000, 0.9238795325112867385, 1.000000000000000000, 0.9238795325112867385, 1.000000000000000000, 0.9238795325112867385, 1.000000000000000000, 0.9238795325112867385, 1.000000000000000000, 0.9238795325112867385, 1.000000000000000000, 0.9238795325112867385, 1.000000000000000000, 0.9238795325112867385, 1.000000000000000000, 0.9238795325112867385, 1.000000000000000000, 0.9238795325112867385, 1.000000000000000000, 0.9238795325112867385, 1.000000000000000000, 0.9238795325112867385, 1.000000000000000000, 0.9238795325112867385, 1.000000000000000000, 0.9238795325112867385, 1.000000000000000000, 0.9238795325112867385, 1.000000000000000000, 0.9238795325112867385, 1.000000000000000000, 0.9238795325112867385, 1.000000000000000000, 0.9238795325112867385, 1.000000000000000000, 0.9238795325112867385, 1.000000000000000000, 0.9238795325112867385, 1.000000000000000000, 0.9238795325112867385, 1.000000000000000000, 0.9238795325112867385, 1.000000000000000000, 0.9238795325112867385, 1.000000000000000000, 0.9238795325112867385, 1.000000000000000000, 0.9238795325112867385, 1.000000000000000000, 0.9238795325112867385, 1.000000000000000000, 0.9238795325112867385, 1.000000000000000000, 0.9238795325112867385, 1.000000000000000000, 0.9238795325112867385, 1.000000000000000000, 0.9238795325112867385, 1.000000000000000000, 0.9238795325112867385, 1.000000000000000000, 0.9238795325112867385, 1.000000000000000000, 0.9238795325112867385, 1.000000000000000000, 0.9238795325112867385, 1.000000000000000000, 0.9238795325112867385, 1.000000000000000000, 0.9238795325112867385, 1.000000000000000000, 0.9238795325112867385, 1.000000000000000000, 0.9238795325112867385, 1.000000000000000000, 0.9238795325112867385, 1.000000000000000000, 0.9238795325112867385, 1.000000000000000000, 0.9238795325112867385, 1.000000000000000000, 0.9238795325112867385, 1.000000000000000000, 0.9238795325112867385, 1.000000000000000000, 0.9238795325112867385, 1.000000000000000000, 0.9238795325112867385, 1.000000000000000000, 0.9238795325112867385, 1.000000000000000000, 0.9238795325112867385, 1.000000000000000000, 0.9238795325112867385, 1.000000000000000000, 0.9238795325112867385, 1.000000000000000000, 0.9238795325112867385, 1.000000000000000000, 0.9238795325112867385, 1.000000000000000000, 0.9238795325112867385, 1.000000000000000000, 0.9238795325112867385, 1.000000000000000000, 0.9238795325112867385, 1.000000000000000000, 0.9238795325112867385, 1.000000000000000000),
 ( 1.000000000000000000, 0.9238795325112867385, 1.000000000000000000, 0.9238795325112867385, 1.000000000000000000, 0.9238795325112867385, 1.000000000000000000, 0.9238795325112867385, 1.000000000000000000, 0.9238795325112867385, 1.000000000000000000, 0.9238795325112867385, 1.000000000000000000, 0.9238795325112867385, 1.000000000000000000, 0.9238795325112867385, 1.000000000000000000, 0.9238795325112867385, 1.000000000000000000, 0.9238795325112867385, 1.000000000000000000, 0.9238795325112867385, 1.000000000000000000, 0.9238795325112867385, 1.000000000000000000, 0.9238795325112867385, 1.000000000000000000, 0.9238795325112867385, 1.000000000000000000, 0.9238795325112867385, 1.000000000000000000, 0.9238795325112867385, 1.000000000000000000, 0.9238795325112867385, 1.000000000000000000, 0.9238795325112867385, 1.000000000000000000, 0.9238795325112867385, 1.000000000000000000, 0.9238795325112867385, 1.000000000000000000, 0.9238795325112867385, 1.000000000000000000, 0.9238795325112867385, 1.000000000000000000, 0.9238795325112867385, 1.000000000000000000, 0.9238795325112867385, 1.000000000000000000, 0.9238795325112867385, 1.000000000000000000, 0.9238795325112867385, 1.000000000000000000, 0.9238795325112867385, 1.000000000000000000, 0.9238795325112867385, 1.000000000000000000, 0.9238795325112867385, 1.000000000000000000, 0.9238795325112867385, 1.000000000000000000, 0.9238795325112867385, 1.000000000000000000, 0.9238795325112867385, 1.000000000000000000, 0.9238795325112867385, 1.000000000000000000, 0.9238795325112867385, 1.000000000000000000, 0.9238795325112867385, 1.000000000000000000, 0.9238795325112867385, 1.000000000000000000, 0.9238795325112867385, 1.000000000000000000, 0.9238795325112867385, 1.000000000000000000, 0.9238795325112867385, 1.000000000000000000, 0.9238795325112867385, 1.000000000000000000, 0.9238795325112867385, 1.000000000000000000, 0.9238795325112867385, 1.000000000000000000, 0.9238795325112867385, 1.000000000000000000, 0.9238795325112867385, 1.000000000000000000, 0.9238795325112867385, 1.000000000000000000, 0.9238795325112867385, 1.000000000000000000, 0.9238795325112867385, 1.000000000000000000, 0.9238795325112867385, 1.000000000000000000, 0.9238795325112867385, 1.000000000000000000, 0.9238795325112867385, 1.000000000000000000, 0.9238795325112867385, 1.000000000000000000, 0.9238795325112867385, 1.000000000000000000, 0.9238795325112867385, 1.000000000000000000, 0.9238795325112867385, 1.000000000000000000, 0.9238795325112867385, 1.000000000000000000, 0.9238795325112867385, 1.000000000000000000, 0.9238795325112867385, 1.000000000000000000, 0.9238795325112867385, 1.000000000000000000, 0.9238795325112867385, 1.000000000000000000, 0.9238795325112867385, 1.000000000000000000, 0.9238795325112867385, 1.000000000000000000, 0.9238795325112867385, 1.000000000000000000, 0.9238795325112867385, 1.000000000000000000, 0.9238795325112867385, 1.000000000000000000, 0.9238795325112867385, 1.000000000000000000, 0.9238795325112867385, 1.000000000000000000, 0.9238795325112867385, 1.000000000000000000, 0.9238795325112867385, 1.000000000000000000, 0.9238795325112867385, 1.000000000000000000, 0.9238795325112867385, 1.000000000000000000, 0.9238795325112867385, 1.000000000000000000, 0.9238795325112867385, 1.000000000000000000, 0.9238795325112867385, 1.000000000000000000, 0.9238795325112867385, 1.000000000000000000) ) ) 
 REPRESENTATION_ITEM ( '' )  SURFACE ( )  );
#18781=CARTESIAN_POINT ( 'NONE',  ( 2.445694354108821411, 2.445694354108820523, 17.06250000136560629 ) ) ;
#18787=CARTESIAN_POINT ( 'NONE',  ( 1.971781867644420635E-15, -4.000000000000000000, 12.25000000000001066 ) ) ;
#18799=CARTESIAN_POINT ( 'NONE',  ( -3.999999999999998224, -1.656854249492383246, 14.06250000000001066 ) ) ;
#18802=CARTESIAN_POINT ( 'NONE',  ( 4.000000000000000888, 1.656854249492381248, 17.68750000273119483 ) ) ;
#18808=CARTESIAN_POINT ( 'NONE',  ( -3.458734124999998993, -1.432654583217642497, 13.50000000136560452 ) ) ;
#18809=LINE ( 'NONE', #5995, #18543 ) ;
#18813=CARTESIAN_POINT ( 'NONE',  ( 1.432654583217641164, 3.458734125000000326, 11.12500000136560452 ) ) ;
#18825=CARTESIAN_POINT ( 'NONE',  ( -3.458734124999999437, 0.000000000000000000, 15.68750000136560629 ) ) ;
#18835=CARTESIAN_POINT ( 'NONE',  ( 3.458734125000001214, 4.235727675282971730E-16, 11.93750000136560629 ) ) ;
#18836=CARTESIAN_POINT ( 'NONE',  ( -2.828427124746188515, -2.828427124746190735, 17.25000000273119838 ) ) ;
#18846=CARTESIAN_POINT ( 'NONE',  ( 4.000000000000000888, 1.656854249492381248, 13.56250000000001066 ) ) ;
#18848=CARTESIAN_POINT ( 'NONE',  ( -3.999999999999999112, 1.656854249492380582, 14.93750000000001066 ) ) ;
#18851=DIRECTION ( 'NONE',  ( -1.000000000000000000, 0.000000000000000000, 0.000000000000000000 ) ) ;
#18855=EDGE_CURVE ( 'NONE', #6890, #14629, #14749, .T. ) ;
#18862=CARTESIAN_POINT ( 'NONE',  ( -2.445694354108818303, -2.445694354108820967, 13.81250000136560629 ) ) ;
#18870=ORIENTED_EDGE ( 'NONE', *, *, #3793, .F. ) ;
#18873=( BOUNDED_CURVE ( )  B_SPLINE_CURVE ( 2, ( #13073, #3934, #11269, #343, #16762, #18544, #2130, #9465, #15107 ),
 .UNSPECIFIED., .F., .F. ) 
 B_SPLINE_CURVE_WITH_KNOTS ( ( 3, 2, 2, 2, 3 ),
 ( 0.2500000000000000000, 0.2625000000000000111, 0.2750000000000000222, 0.2874999999999999778, 0.2999999999999999889 ),
 .UNSPECIFIED. ) 
 CURVE ( )  GEOMETRIC_REPRESENTATION_ITEM ( )  RATIONAL_B_SPLINE_CURVE ( ( 1.000000000000000000, 0.9238795325112867385, 1.000000000000000000, 0.9238795325112867385, 1.000000000000000000, 0.9238795325112867385, 1.000000000000000000, 0.9238795325112867385, 1.000000000000000000 ) ) 
 REPRESENTATION_ITEM ( '' )  );
#18875=ORIENTED_EDGE ( 'NONE', *, *, #2134, .F. ) ;
#18879=EDGE_CURVE ( 'NONE', #3586, #9317, #786, .T. ) ;
#18882=ADVANCED_FACE ( 'NONE', ( #19106 ), #2697, .F. ) ;
#18894=PLANE ( 'NONE',  #10748 ) ;
#18901=CARTESIAN_POINT ( 'NONE',  ( 1.971781867644420635E-15, -4.000000000000000000, 11.37500000273119660 ) ) ;
#18907=CARTESIAN_POINT ( 'NONE',  ( -2.828427124746188515, -2.828427124746190735, 15.12500000000001066 ) ) ;
#18917=CARTESIAN_POINT ( 'NONE',  ( 2.445694354108821855, -2.445694354108820079, 12.81250000136560629 ) ) ;
#18927=CARTESIAN_POINT ( 'NONE',  ( 2.445694354108821411, 2.445694354108820523, 11.06250000136560452 ) ) ;
#18929=ORIENTED_EDGE ( 'NONE', *, *, #9100, .T. ) ;
#18939=CARTESIAN_POINT ( 'NONE',  ( 2.445694354108821411, 2.445694354108820523, 18.31250000136560274 ) ) ;
#18947=CARTESIAN_POINT ( 'NONE',  ( -15.00000000000000711, 10.00000000000000000, -19.99999999999999645 ) ) ;
#18949=CARTESIAN_POINT ( 'NONE',  ( -1.432654583217638944, 3.458734125000000326, 11.25000000136560452 ) ) ;
#18950=CARTESIAN_POINT ( 'NONE',  ( 1.656854249492384135, -3.999999999999999112, 11.43750000273119660 ) ) ;
#18961=ORIENTED_EDGE ( 'NONE', *, *, #21834, .T. ) ;
#18962=CARTESIAN_POINT ( 'NONE',  ( -1.656854249492379250, 4.000000000000000000, 14.81250000000001066 ) ) ;
#18970=CARTESIAN_POINT ( 'NONE',  ( 1.432654583217641386, 3.458734125000000770, 18.37500000136560629 ) ) ;
#18976=CARTESIAN_POINT ( 'NONE',  ( -2.445694354108818303, -2.445694354108820967, 10.81250000136560452 ) ) ;
#18980=ORIENTED_EDGE ( 'NONE', *, *, #22727, .F. ) ;
#19000=CARTESIAN_POINT ( 'NONE',  ( -3.458734124999998105, -1.432654583217642275, 18.50000000136560629 ) ) ;
#19012=DIRECTION ( 'NONE',  ( -0.000000000000000000, 1.000000000000000000, -0.000000000000000000 ) ) ;
#19017=CARTESIAN_POINT ( 'NONE',  ( -20.00000000000000711, 9.999999999999964473, -19.99999999999999645 ) ) ;
#19019=CARTESIAN_POINT ( 'NONE',  ( 9.920644283265380691E-16, 4.000000000000000000, 17.75000000000000711 ) ) ;
#19027=ADVANCED_BREP_SHAPE_REPRESENTATION ( '', ( #21929, #7318 ), #13013 ) ;
#19028=LINE ( 'NONE', #4658, #12188 ) ;
#19033=CARTESIAN_POINT ( 'NONE',  ( 4.000000000000001776, -1.656854249492379694, 10.56250000273119660 ) ) ;
#19035=CARTESIAN_POINT ( 'NONE',  ( 1.432654583217643163, -3.458734124999999437, 13.75000000136560452 ) ) ;
#19041=CARTESIAN_POINT ( 'NONE',  ( -3.458734124999998993, -1.432654583217642497, 11.50000000136560629 ) ) ;
#19043=ORIENTED_EDGE ( 'NONE', *, *, #110, .T. ) ;
#19044=AXIS2_PLACEMENT_3D ( 'NONE', #19984, #3587, #10925 ) ;
#19057=CARTESIAN_POINT ( 'NONE',  ( -1.432654583217639166, 3.458734125000000770, 17.50000000136560274 ) ) ;
#19068=AXIS2_PLACEMENT_3D ( 'NONE', #21509, #17480, #3089 ) ;
#19071=CARTESIAN_POINT ( 'NONE',  ( -1.656854249492380138, -3.999999999999999112, 10.31250000273119483 ) ) ;
#19073=ORIENTED_EDGE ( 'NONE', *, *, #10920, .T. ) ;
#19093=CARTESIAN_POINT ( 'NONE',  ( 1.432654583217641386, 3.458734125000000770, 19.37500000136560629 ) ) ;
#19098=CARTESIAN_POINT ( 'NONE',  ( -7.229187218286264707E-16, 1.417950490603859619E-15, 10.00000000000000888 ) ) ;
#19101=CARTESIAN_POINT ( 'NONE',  ( -3.458734124999998993, -1.432654583217642497, 12.75000000136560629 ) ) ;
#19106=FACE_OUTER_BOUND ( 'NONE', #12209, .T. ) ;
#19107=ORIENTED_EDGE ( 'NONE', *, *, #23257, .F. ) ;
#19126=CARTESIAN_POINT ( 'NONE',  ( 4.000000000000000888, 4.898587196589412829E-16, 14.62500000273119660 ) ) ;
#19128=CARTESIAN_POINT ( 'NONE',  ( 1.656854249492384135, -3.999999999999999112, 12.43750000273119838 ) ) ;
#19129=CARTESIAN_POINT ( 'NONE',  ( 2.445694354108821855, -2.445694354108820079, 17.81250000136560274 ) ) ;
#19134=ADVANCED_FACE ( 'NONE', ( #7606 ), #44, .T. ) ;
#19145=CARTESIAN_POINT ( 'NONE',  ( 9.920644283265380691E-16, 4.000000000000000000, 10.75000000000001066 ) ) ;
#19157=CARTESIAN_POINT ( 'NONE',  ( 3.458734125000001214, 4.235727675282971730E-16, 11.93750000136560629 ) ) ;
#19168=CARTESIAN_POINT ( 'NONE',  ( 14.99999999999995737, -15.00000000000000000, -50.00000000000000000 ) ) ;
#19172=EDGE_LOOP ( 'NONE', ( #17157, #21759, #15915, #21296 ) ) ;
#19177=CARTESIAN_POINT ( 'NONE',  ( 1.872352939448454495E-15, -3.458734125000000770, 14.93750000136560452 ) ) ;
#19189=CARTESIAN_POINT ( 'NONE',  ( 1.656854249492381470, 4.000000000000000000, 13.81250000273119483 ) ) ;
#19208=CARTESIAN_POINT ( 'NONE',  ( -3.999999999999999112, 0.000000000000000000, 15.00000000000001066 ) ) ;
#19209=CARTESIAN_POINT ( 'NONE',  ( -3.458734124999999437, 1.432654583217640498, 18.62500000136560629 ) ) ;
#19210=CARTESIAN_POINT ( 'NONE',  ( 4.000000000000000888, 1.656854249492381248, 13.68750000273119483 ) ) ;
#19216=CARTESIAN_POINT ( 'NONE',  ( 3.458734125000001658, 4.235727675282972223E-16, 11.18750000136560452 ) ) ;
#19231=CARTESIAN_POINT ( 'NONE',  ( 27.50000000000000000, 7.500000000000001776, -33.66025403784446723 ) ) ;
#19239=CARTESIAN_POINT ( 'NONE',  ( 1.025207404391860050E-15, 3.458734125000000326, 19.18750000136560629 ) ) ;
#19249=CARTESIAN_POINT ( 'NONE',  ( 2.828427124746192067, -2.828427124746189847, 11.50000000273119660 ) ) ;
#19259=CARTESIAN_POINT ( 'NONE',  ( -2.828427124746188515, -2.828427124746190735, 16.12500000000001066 ) ) ;
#19263=DIRECTION ( 'NONE',  ( -1.224646799147353207E-16, 0.000000000000000000, -1.000000000000000000 ) ) ;
#19264=CARTESIAN_POINT ( 'NONE',  ( -3.999999999999998224, -1.656854249492383024, 10.18750000273119660 ) ) ;
#19266=CARTESIAN_POINT ( 'NONE',  ( 3.458734125000001658, 1.432654583217640498, 17.25000000136560629 ) ) ;
#19274=ORIENTED_EDGE ( 'NONE', *, *, #14442, .T. ) ;
#19281=ADVANCED_FACE ( 'NONE', ( #20741 ), #9756, .T. ) ;
#19284=CARTESIAN_POINT ( 'NONE',  ( 1.432654583217643163, -3.458734124999999882, 14.00000000136560629 ) ) ;
#19297=CARTESIAN_POINT ( 'NONE',  ( 1.971781867644420635E-15, -4.000000000000000000, 12.37500000273119838 ) ) ;
#19299=VERTEX_POINT ( 'NONE', #4347 ) ;
#19305=ORIENTED_EDGE ( 'NONE', *, *, #7667, .F. ) ;
#19311=DIRECTION ( 'NONE',  ( -0.3373062947069096484, 0.9413949561959079615, 0.000000000000000000 ) ) ;
#19315=EDGE_CURVE ( 'NONE', #13219, #19809, #17068, .T. ) ;
#19319=CARTESIAN_POINT ( 'NONE',  ( -2.445694354108819191, 2.445694354108820523, 18.56250000136560629 ) ) ;
#19320=CARTESIAN_POINT ( 'NONE',  ( 2.828427124746192067, -2.828427124746189847, 15.50000000273119660 ) ) ;
#19335=CARTESIAN_POINT ( 'NONE',  ( -1.656854249492380138, -3.999999999999999112, 15.31250000273119660 ) ) ;
#19343=CARTESIAN_POINT ( 'NONE',  ( 1.236993788156008760E-15, 0.000000000000000000, 21.31370849898476649 ) ) ;
#19346=EDGE_CURVE ( 'NONE', #9768, #21282, #8832, .T. ) ;
#19350=( BOUNDED_CURVE ( )  B_SPLINE_CURVE ( 2, ( #15726, #22996, #6602, #13920, #21175, #19388, #17628, #21289, #4912 ),
 .UNSPECIFIED., .F., .F. ) 
 B_SPLINE_CURVE_WITH_KNOTS ( ( 3, 2, 2, 2, 3 ),
 ( 0.5500000000000000444, 0.5625000000000000000, 0.5749999999999999556, 0.5875000000000000222, 0.5999999999999999778 ),
 .UNSPECIFIED. ) 
 CURVE ( )  GEOMETRIC_REPRESENTATION_ITEM ( )  RATIONAL_B_SPLINE_CURVE ( ( 1.000000000000000000, 0.9238795325112867385, 1.000000000000000000, 0.9238795325112867385, 1.000000000000000000, 0.9238795325112867385, 1.000000000000000000, 0.9238795325112867385, 1.000000000000000000 ) ) 
 REPRESENTATION_ITEM ( '' )  );
#19353=CARTESIAN_POINT ( 'NONE',  ( -2.445694354108819191, 2.445694354108820523, 13.31250000136560452 ) ) ;
#19356=ORIENTED_EDGE ( 'NONE', *, *, #13918, .T. ) ;
#19366=DIRECTION ( 'NONE',  ( 0.000000000000000000, -1.000000000000000000, 0.000000000000000000 ) ) ;
#19367=ADVANCED_FACE ( 'NONE', ( #14297 ), #12387, .F. ) ;
#19370=CARTESIAN_POINT ( 'NONE',  ( 1.971781867644420635E-15, -4.000000000000000000, 19.25000000000001066 ) ) ;
#19371=CARTESIAN_POINT ( 'NONE',  ( 2.828427124746191179, 2.828427124746190291, 11.62500000000001066 ) ) ;
#19377=CARTESIAN_POINT ( 'NONE',  ( -1.432654583217639166, 3.458734125000000770, 19.50000000136560629 ) ) ;
#19383=CARTESIAN_POINT ( 'NONE',  ( 2.828427124746191179, 2.828427124746190291, 15.62500000000001066 ) ) ;
#19385=DIRECTION ( 'NONE',  ( -0.9413949561959078505, -0.3373062947069098150, 1.152876319838781169E-16 ) ) ;
#19388=CARTESIAN_POINT ( 'NONE',  ( -1.656854249492380138, -3.999999999999999112, 13.31250000273119660 ) ) ;
#19394=DIRECTION ( 'NONE',  ( 0.000000000000000000, -1.000000000000000000, 0.000000000000000000 ) ) ;
#19395=ORIENTED_EDGE ( 'NONE', *, *, #23128, .T. ) ;
#19398=CARTESIAN_POINT ( 'NONE',  ( 1.432654583217641386, 3.458734125000000770, 11.37500000136560452 ) ) ;
#19407=EDGE_CURVE ( 'NONE', #17227, #19630, #4938, .T. ) ;
#19411=CARTESIAN_POINT ( 'NONE',  ( -2.828427124746189403, 2.828427124746190291, 12.00000000273119660 ) ) ;
#19420=EDGE_CURVE ( 'NONE', #16157, #13512, #9444, .T. ) ;
#19431=DIRECTION ( 'NONE',  ( 0.000000000000000000, 0.000000000000000000, 1.000000000000000000 ) ) ;
#19436=CARTESIAN_POINT ( 'NONE',  ( 3.458734125000001658, 4.235727675282972223E-16, 16.18750000136560629 ) ) ;
#19437=CARTESIAN_POINT ( 'NONE',  ( 4.000000000000000888, 1.656854249492381248, 12.68750000273119660 ) ) ;
#19459=EDGE_CURVE ( 'NONE', #17446, #4526, #7077, .T. ) ;
#19466=CARTESIAN_POINT ( 'NONE',  ( 1.656854249492381470, 4.000000000000000000, 11.68750000000001066 ) ) ;
#19475=EDGE_CURVE ( 'NONE', #13926, #17599, #7928, .T. ) ;
#19477=CARTESIAN_POINT ( 'NONE',  ( 1.872352939448454495E-15, -3.458734125000000326, 16.68750000136560629 ) ) ;
#19487=DIRECTION ( 'NONE',  ( 0.000000000000000000, 0.000000000000000000, 1.000000000000000000 ) ) ;
#19505=CARTESIAN_POINT ( 'NONE',  ( 1.872352939448454495E-15, -3.458734125000000770, 18.93750000136560629 ) ) ;
#19507=CARTESIAN_POINT ( 'NONE',  ( 4.000000000000000888, 4.898587196589412829E-16, 15.50000000000001066 ) ) ;
#19513=DIRECTION ( 'NONE',  ( -0.000000000000000000, -1.000000000000000000, 0.000000000000000000 ) ) ;
#19521=CARTESIAN_POINT ( 'NONE',  ( -2.828427124746189403, 2.828427124746190291, 13.00000000273119660 ) ) ;
#19523=CARTESIAN_POINT ( 'NONE',  ( -3.458734124999999437, 0.000000000000000000, 11.68750000136560629 ) ) ;
#19532=( BOUNDED_CURVE ( )  B_SPLINE_CURVE ( 2, ( #14108, #12560, #8487, #8844, #12201, #23062, #19585, #23542, #3426 ),
 .UNSPECIFIED., .F., .F. ) 
 B_SPLINE_CURVE_WITH_KNOTS ( ( 3, 2, 2, 2, 3 ),
 ( 0.1499999999999999944, 0.1625000000000000056, 0.1749999999999999889, 0.1875000000000000000, 0.2000000000000000111 ),
 .UNSPECIFIED. ) 
 CURVE ( )  GEOMETRIC_REPRESENTATION_ITEM ( )  RATIONAL_B_SPLINE_CURVE ( ( 1.000000000000000000, 0.9238795325112867385, 1.000000000000000000, 0.9238795325112867385, 1.000000000000000000, 0.9238795325112867385, 1.000000000000000000, 0.9238795325112867385, 1.000000000000000000 ) ) 
 REPRESENTATION_ITEM ( '' )  );
#19534=DIRECTION ( 'NONE',  ( -0.000000000000000000, -0.000000000000000000, -1.000000000000000000 ) ) ;
#19536=CARTESIAN_POINT ( 'NONE',  ( 2.445694354108821855, -2.445694354108820079, 15.81250000136560629 ) ) ;
#19540=CARTESIAN_POINT ( 'NONE',  ( 1.971781867644420635E-15, -4.000000000000000000, 14.37500000273119660 ) ) ;
#19552=EDGE_CURVE ( 'NONE', #21603, #2255, #11137, .T. ) ;
#19555=CARTESIAN_POINT ( 'NONE',  ( 1.432654583217643163, -3.458734124999999882, 17.00000000136560629 ) ) ;
#19556=CARTESIAN_POINT ( 'NONE',  ( -3.999999999999999112, 1.656854249492380804, 10.06250000273119660 ) ) ;
#19559=CARTESIAN_POINT ( 'NONE',  ( 4.000000000000000888, 4.898587196589412829E-16, 17.62500000273119483 ) ) ;
#19564=ORIENTED_EDGE ( 'NONE', *, *, #12329, .F. ) ;
#19571=ORIENTED_EDGE ( 'NONE', *, *, #4507, .T. ) ;
#19574=DIRECTION ( 'NONE',  ( 1.000000000000000000, 0.000000000000000000, 0.000000000000000000 ) ) ;
#19576=DIRECTION ( 'NONE',  ( 1.000000000000000000, 0.000000000000000000, 0.000000000000000000 ) ) ;
#19585=CARTESIAN_POINT ( 'NONE',  ( -2.828427124746188515, -2.828427124746190735, 17.25000000273119838 ) ) ;
#19586=CYLINDRICAL_SURFACE ( 'NONE', #16073, 4.999999999999999112 ) ;
#19589=CARTESIAN_POINT ( 'NONE',  ( 3.458734125000001214, 1.432654583217640498, 15.00000000136560807 ) ) ;
#19590=CARTESIAN_POINT ( 'NONE',  ( -0.8800590352214044954, 5.420839058164813373, -19.99999999999999645 ) ) ;
#19600=CARTESIAN_POINT ( 'NONE',  ( 4.000000000000000888, 4.898587196589412829E-16, 16.50000000000001066 ) ) ;
#19616=CARTESIAN_POINT ( 'NONE',  ( 1.432654583217641386, 3.458734125000000770, 18.37500000136560274 ) ) ;
#19629=VECTOR ( 'NONE', #7639, 1000.000000000000000 ) ;
#19630=VERTEX_POINT ( 'NONE', #2983 ) ;
#19633=CARTESIAN_POINT ( 'NONE',  ( 1.656854249492381470, 4.000000000000000000, 12.81250000273119660 ) ) ;
#19634=( BOUNDED_CURVE ( )  B_SPLINE_CURVE ( 2, ( #17064, #18848, #16947, #15055, #15408, #17187, #22310, #11812, #13252 ),
 .UNSPECIFIED., .F., .F. ) 
 B_SPLINE_CURVE_WITH_KNOTS ( ( 3, 2, 2, 2, 3 ),
 ( 0.5000000000000000000, 0.5124999999999999556, 0.5250000000000000222, 0.5374999999999999778, 0.5500000000000000444 ),
 .UNSPECIFIED. ) 
 CURVE ( )  GEOMETRIC_REPRESENTATION_ITEM ( )  RATIONAL_B_SPLINE_CURVE ( ( 1.000000000000000000, 0.9238795325112867385, 1.000000000000000000, 0.9238795325112867385, 1.000000000000000000, 0.9238795325112867385, 1.000000000000000000, 0.9238795325112867385, 1.000000000000000000 ) ) 
 REPRESENTATION_ITEM ( '' )  );
#19636=CARTESIAN_POINT ( 'NONE',  ( -2.828427124746189403, 2.828427124746190291, 17.87500000000001066 ) ) ;
#19644=CARTESIAN_POINT ( 'NONE',  ( 4.000000000000000888, 4.898587196589412829E-16, 14.50000000000001066 ) ) ;
#19649=CARTESIAN_POINT ( 'NONE',  ( 1.872352939448454495E-15, -3.458734125000000326, 18.68750000136560629 ) ) ;
#19652=CARTESIAN_POINT ( 'NONE',  ( 14.99999999999995559, -15.00000000000000000, -50.00000000000000000 ) ) ;
#19665=AXIS2_PLACEMENT_3D ( 'NONE', #3990, #13239, #9525 ) ;
#19669=CARTESIAN_POINT ( 'NONE',  ( -1.432654583217639166, 3.458734125000000770, 16.50000000136560629 ) ) ;
#19677=EDGE_CURVE ( 'NONE', #21587, #22281, #19350, .T. ) ;
#19679=CARTESIAN_POINT ( 'NONE',  ( 27.50000000000000000, 7.500000000000001776, -31.01025403784447221 ) ) ;
#19691=VERTEX_POINT ( 'NONE', #8637 ) ;
#19692=SURFACE_STYLE_USAGE ( .BOTH. , #21130 ) ;
#19699=FACE_OUTER_BOUND ( 'NONE', #21385, .T. ) ;
#19703=CARTESIAN_POINT ( 'NONE',  ( -3.458734124999998993, 0.000000000000000000, 16.43750000136560629 ) ) ;
#19713=ORIENTED_EDGE ( 'NONE', *, *, #8366, .F. ) ;
#19728=CARTESIAN_POINT ( 'NONE',  ( -3.999999999999999112, 0.000000000000000000, 21.31370849898476649 ) ) ;
#19730=DIRECTION ( 'NONE',  ( 0.000000000000000000, 0.000000000000000000, 1.000000000000000000 ) ) ;
#19734=DIRECTION ( 'NONE',  ( 1.224646799147353207E-16, 0.000000000000000000, 1.000000000000000000 ) ) ;
#19735=CARTESIAN_POINT ( 'NONE',  ( -3.458734124999999437, 1.432654583217640498, 17.62500000136560274 ) ) ;
#19751=ORIENTED_EDGE ( 'NONE', *, *, #15839, .T. ) ;
#19755=CARTESIAN_POINT ( 'NONE',  ( 1.656854249492384135, -3.999999999999999112, 19.31250000000001776 ) ) ;
#19757=CARTESIAN_POINT ( 'NONE',  ( -1.656854249492379472, 4.000000000000000000, 10.81250000000001243 ) ) ;
#19768=CARTESIAN_POINT ( 'NONE',  ( 3.458734125000002102, -1.432654583217639610, 16.87500000136560629 ) ) ;
#19773=ORIENTED_EDGE ( 'NONE', *, *, #14484, .F. ) ;
#19785=ORIENTED_EDGE ( 'NONE', *, *, #9977, .F. ) ;
#19791=CARTESIAN_POINT ( 'NONE',  ( 1.025207404391860050E-15, 3.458734125000000770, 17.43750000136560274 ) ) ;
#19792=CARTESIAN_POINT ( 'NONE',  ( 9.920644283265380691E-16, 4.000000000000000000, 9.875000002731196602 ) ) ;
#19794=VECTOR ( 'NONE', #17910, 1000.000000000000114 ) ;
#19799=CARTESIAN_POINT ( 'NONE',  ( -1.656854249492379250, 4.000000000000000000, 18.93750000273119838 ) ) ;
#19809=VERTEX_POINT ( 'NONE', #3929 ) ;
#19810=CARTESIAN_POINT ( 'NONE',  ( -1.656854249492380138, -3.999999999999999112, 19.18750000000001066 ) ) ;
#19811=ORIENTED_EDGE ( 'NONE', *, *, #4539, .F. ) ;
#19815=CARTESIAN_POINT ( 'NONE',  ( 19.99999999999998934, -9.999999999999964473, -50.00000000000000000 ) ) ;
#19825=CARTESIAN_POINT ( 'NONE',  ( 1.432654583217641164, 3.458734125000000326, 14.12500000136560452 ) ) ;
#19828=ORIENTED_EDGE ( 'NONE', *, *, #3203, .F. ) ;
#19834=ORIENTED_EDGE ( 'NONE', *, *, #8664, .F. ) ;
#19850=ORIENTED_EDGE ( 'NONE', *, *, #12050, .T. ) ;
#19851=CARTESIAN_POINT ( 'NONE',  ( 1.971781867644420635E-15, -4.000000000000000000, 18.37500000273119483 ) ) ;
#19860=DIRECTION ( 'NONE',  ( 0.9413949561959078505, 0.3373062947069098150, 0.000000000000000000 ) ) ;
#19862=CYLINDRICAL_SURFACE ( 'NONE', #14682, 4.000000000000000000 ) ;
#19875=CARTESIAN_POINT ( 'NONE',  ( 4.000000000000000888, 1.656854249492381248, 19.56250000000001421 ) ) ;
#19892=CARTESIAN_POINT ( 'NONE',  ( 1.432654583217641164, 3.458734125000000326, 18.12500000136560274 ) ) ;
#19901=ORIENTED_EDGE ( 'NONE', *, *, #1236, .T. ) ;
#19902=VECTOR ( 'NONE', #8034, 1000.000000000000000 ) ;
#19910=CARTESIAN_POINT ( 'NONE',  ( -3.458734124999998105, -1.432654583217642497, 13.75000000136560452 ) ) ;
#19911=CARTESIAN_POINT ( 'NONE',  ( -3.999999999999998224, -1.656854249492383246, 11.18750000273119660 ) ) ;
#19916=EDGE_CURVE ( 'NONE', #10729, #12579, #16999, .T. ) ;
#19927=CARTESIAN_POINT ( 'NONE',  ( -27.50000000000000711, 7.500000000000001776, -36.31025403784445871 ) ) ;
#19929=CARTESIAN_POINT ( 'NONE',  ( -3.999999999999999112, 0.000000000000000000, 19.00000000000001066 ) ) ;
#19934=( NAMED_UNIT ( * ) SI_UNIT ( $, .STERADIAN. ) SOLID_ANGLE_UNIT ( ) );
#19945=CARTESIAN_POINT ( 'NONE',  ( -1.432654583217639610, -3.458734124999999882, 12.62500000136560629 ) ) ;
#19956=VERTEX_POINT ( 'NONE', #20566 ) ;
#19965=CARTESIAN_POINT ( 'NONE',  ( -1.656854249492380138, -3.999999999999999112, 17.31250000273119483 ) ) ;
#19966=CARTESIAN_POINT ( 'NONE',  ( -2.247776618166720475, 3.308700692843488333, 9.970592379354943802 ) ) ;
#19984=CARTESIAN_POINT ( 'NONE',  ( -15.00000000000001066, -10.00000000000000000, -49.99999999999999289 ) ) ;
#19985=CARTESIAN_POINT ( 'NONE',  ( -2.445694354108818303, -2.445694354108820967, 10.81250000136560452 ) ) ;
#19988=CARTESIAN_POINT ( 'NONE',  ( 19.99999999999998934, 9.999999999999966249, -50.00000000000000000 ) ) ;
#19991=AXIS2_PLACEMENT_3D ( 'NONE', #18947, #6507, #13827 ) ;
#19993=CARTESIAN_POINT ( 'NONE',  ( -2.445694354108818303, -2.445694354108820523, 17.56250000136560274 ) ) ;
#19997=CARTESIAN_POINT ( 'NONE',  ( -3.458734124999998993, -1.432654583217642497, 12.50000000136560452 ) ) ;
#20016=CARTESIAN_POINT ( 'NONE',  ( 2.445694354108821411, 2.445694354108820523, 12.31250000136560629 ) ) ;
#20017=CARTESIAN_POINT ( 'NONE',  ( 1.656854249492384135, -3.999999999999999112, 11.43750000273119660 ) ) ;
#20027=EDGE_LOOP ( 'NONE', ( #12250, #17629, #19751, #8290, #2000, #1516, #5553, #20033 ) ) ;
#20033=ORIENTED_EDGE ( 'NONE', *, *, #13087, .F. ) ;
#20034=CARTESIAN_POINT ( 'NONE',  ( 1.656854249492381470, 4.000000000000000000, 16.68750000000001066 ) ) ;
#20058=ORIENTED_EDGE ( 'NONE', *, *, #15381, .F. ) ;
#20060=CARTESIAN_POINT ( 'NONE',  ( 35.00000000000000000, 4.500000000000001776, -20.00000000000000355 ) ) ;
#20077=CARTESIAN_POINT ( 'NONE',  ( -3.999999999999999112, 0.000000000000000000, 17.12500000273119838 ) ) ;
#20086=FACE_OUTER_BOUND ( 'NONE', #13768, .T. ) ;
#20093=EDGE_CURVE ( 'NONE', #17601, #22004, #16002, .T. ) ;
#20099=CARTESIAN_POINT ( 'NONE',  ( -1.656854249492380138, -3.999999999999999112, 19.18750000000001066 ) ) ;
#20100=LINE ( 'NONE', #16769, #13819 ) ;
#20101=DIRECTION ( 'NONE',  ( -0.000000000000000000, 1.000000000000000000, -0.000000000000000000 ) ) ;
#20106=CARTESIAN_POINT ( 'NONE',  ( 1.025207404391860050E-15, 3.458734125000000326, 16.18750000136560629 ) ) ;
#20111=CARTESIAN_POINT ( 'NONE',  ( -3.458734124999998993, 1.432654583217640276, 13.37500000136560452 ) ) ;
#20128=CARTESIAN_POINT ( 'NONE',  ( -1.432654583217639166, 3.458734125000000770, 12.50000000136560629 ) ) ;
#20133=CARTESIAN_POINT ( 'NONE',  ( 4.000000000000000888, 4.898587196589412829E-16, 16.62500000273119838 ) ) ;
#20134=ADVANCED_FACE ( 'NONE', ( #16235 ), #23646, .T. ) ;
#20141=EDGE_LOOP ( 'NONE', ( #5669, #11937, #20216, #18875 ) ) ;
#20147=CARTESIAN_POINT ( 'NONE',  ( 4.000000000000001776, -1.656854249492379694, 15.43750000000001066 ) ) ;
#20149=AXIS2_PLACEMENT_3D ( 'NONE', #10849, #15876, #18125 ) ;
#20165=CARTESIAN_POINT ( 'NONE',  ( 2.445694354108821411, 2.445694354108820523, 16.31250000136560629 ) ) ;
#20180=DIRECTION ( 'NONE',  ( 1.224646799147353207E-16, 0.000000000000000000, 1.000000000000000000 ) ) ;
#20187=VECTOR ( 'NONE', #7215, 1000.000000000000000 ) ;
#20190=EDGE_CURVE ( 'NONE', #14136, #16438, #9774, .T. ) ;
#20193=CARTESIAN_POINT ( 'NONE',  ( -2.828427124746188515, -2.828427124746190735, 16.25000000273119838 ) ) ;
#20202=EDGE_CURVE ( 'NONE', #2992, #21075, #7382, .T. ) ;
#20212=CARTESIAN_POINT ( 'NONE',  ( -3.999999999999999112, 0.000000000000000000, 15.12500000273119660 ) ) ;
#20216=ORIENTED_EDGE ( 'NONE', *, *, #4730, .F. ) ;
#20219=CARTESIAN_POINT ( 'NONE',  ( -3.999999999999999112, 1.656854249492380804, 13.93750000000001243 ) ) ;
#20231=CARTESIAN_POINT ( 'NONE',  ( -1.432654583217639610, -3.458734124999999882, 17.62500000136560274 ) ) ;
#20235=( GEOMETRIC_REPRESENTATION_CONTEXT ( 3 ) GLOBAL_UNCERTAINTY_ASSIGNED_CONTEXT ( ( #13873 ) ) GLOBAL_UNIT_ASSIGNED_CONTEXT ( ( #7380, #18247, #16122 ) ) REPRESENTATION_CONTEXT ( 'NONE', 'WORKASPACE' ) );
#20239=CARTESIAN_POINT ( 'NONE',  ( 3.458734125000002102, -1.432654583217639610, 11.87500000136560452 ) ) ;
#20241=ORIENTED_EDGE ( 'NONE', *, *, #15381, .T. ) ;
#20248=CARTESIAN_POINT ( 'NONE',  ( -3.999999999999999112, 0.000000000000000000, 17.00000000000001066 ) ) ;
#20251=ORIENTED_EDGE ( 'NONE', *, *, #8131, .F. ) ;
#20257=( BOUNDED_CURVE ( )  B_SPLINE_CURVE ( 2, ( #18226, #18351, #22159, #1809, #18464, #9157, #22033, #5648, #20248 ),
 .UNSPECIFIED., .F., .F. ) 
 B_SPLINE_CURVE_WITH_KNOTS ( ( 3, 2, 2, 2, 3 ),
 ( 0.2500000000000000000, 0.2625000000000000111, 0.2750000000000000222, 0.2874999999999999778, 0.2999999999999999889 ),
 .UNSPECIFIED. ) 
 CURVE ( )  GEOMETRIC_REPRESENTATION_ITEM ( )  RATIONAL_B_SPLINE_CURVE ( ( 1.000000000000000000, 0.9238795325112867385, 1.000000000000000000, 0.9238795325112867385, 1.000000000000000000, 0.9238795325112867385, 1.000000000000000000, 0.9238795325112867385, 1.000000000000000000 ) ) 
 REPRESENTATION_ITEM ( '' )  );
#20258=CARTESIAN_POINT ( 'NONE',  ( 1.432654583217641386, 3.458734125000000770, 13.37500000136560274 ) ) ;
#20264=CARTESIAN_POINT ( 'NONE',  ( -3.999999999999998224, -1.656854249492383246, 15.18750000273119660 ) ) ;
#20267=ORIENTED_EDGE ( 'NONE', *, *, #22089, .T. ) ;
#20276=CARTESIAN_POINT ( 'NONE',  ( -3.999999999999998224, -1.656854249492383246, 17.06250000000001421 ) ) ;
#20290=CARTESIAN_POINT ( 'NONE',  ( 1.872352939448454495E-15, -3.458734125000000770, 15.93750000136560629 ) ) ;
#20298=EDGE_LOOP ( 'NONE', ( #9702, #20836, #54, #21913 ) ) ;
#20312=CARTESIAN_POINT ( 'NONE',  ( -3.999999999999999112, -1.132742959800665972, 19.16772943110984428 ) ) ;
#20313=LINE ( 'NONE', #20554, #23684 ) ;
#20335=CARTESIAN_POINT ( 'NONE',  ( 9.920644283265380691E-16, 4.000000000000000000, 13.75000000000001066 ) ) ;
#20342=LINE ( 'NONE', #11763, #9163 ) ;
#20347=CARTESIAN_POINT ( 'NONE',  ( 2.445694354108821411, 2.445694354108820523, 18.06250000136560274 ) ) ;
#20352=CARTESIAN_POINT ( 'NONE',  ( -3.458734124999998993, -1.432654583217642497, 15.50000000136560807 ) ) ;
#20353=FACE_OUTER_BOUND ( 'NONE', #23441, .T. ) ;
#20361=ORIENTED_EDGE ( 'NONE', *, *, #18879, .T. ) ;
#20364=CARTESIAN_POINT ( 'NONE',  ( -3.458734124999999437, 0.000000000000000000, 17.68750000136560274 ) ) ;
#20378=CARTESIAN_POINT ( 'NONE',  ( -2.445694354108818303, -2.445694354108820523, 12.56250000136560629 ) ) ;
#20379=CARTESIAN_POINT ( 'NONE',  ( -3.999999999999999112, 1.656854249492380804, 15.06250000273119483 ) ) ;
#20391=CARTESIAN_POINT ( 'NONE',  ( -1.656854249492379250, 4.000000000000000000, 12.81250000000001066 ) ) ;
#20396=CLOSED_SHELL ( 'NONE', ( #9136, #21923, #13344, #16131, #20134, #819, #7166, #14976, #706, #82, #15101, #18551, #19134, #1362, #7349, #23421, #14677, #21093, #10580, #21896, #8761, #21298, #10768, #11931, #16380, #22365, #16684, #2022, #171, #7056, #14539, #11402, #3958, #19281, #19367, #16153, #11748, #6470, #3505, #14704, #23063, #11165, #9832, #781, #14032, #8537, #2162, #2309, #18882, #22057, #14648, #6293, #21098, #1699 ) ) ;
#20403=CARTESIAN_POINT ( 'NONE',  ( 9.920644283265380691E-16, 4.000000000000000000, 9.875000002731196602 ) ) ;
#20406=CARTESIAN_POINT ( 'NONE',  ( -2.445694354108818303, -2.445694354108820967, 16.81250000136560629 ) ) ;
#20425=CARTESIAN_POINT ( 'NONE',  ( 4.000000000000000888, 4.898587196589412829E-16, 21.31370849898476649 ) ) ;
#20429=CARTESIAN_POINT ( 'NONE',  ( 4.000000000000001776, -1.656854249492379694, 15.56250000273119660 ) ) ;
#20445=ORIENTED_EDGE ( 'NONE', *, *, #3105, .F. ) ;
#20446=CARTESIAN_POINT ( 'NONE',  ( -35.00000000000000711, 7.500000000000001776, -49.99999999999998579 ) ) ;
#20455=FACE_OUTER_BOUND ( 'NONE', #16614, .T. ) ;
#20456=CARTESIAN_POINT ( 'NONE',  ( -1.656854249492379250, 4.000000000000000000, 13.81250000000001066 ) ) ;
#20461=VERTEX_POINT ( 'NONE', #15862 ) ;
#20466=CARTESIAN_POINT ( 'NONE',  ( 4.000000000000000888, 4.898587196589412829E-16, 11.62500000273119660 ) ) ;
#20468=CARTESIAN_POINT ( 'NONE',  ( 1.872352939448454495E-15, -3.458734125000000326, 18.68750000136560629 ) ) ;
#20473=CARTESIAN_POINT ( 'NONE',  ( 2.445694354108821411, 2.445694354108820523, 15.06250000136560452 ) ) ;
#20490=CARTESIAN_POINT ( 'NONE',  ( 2.445694354108821411, 2.445694354108820523, 15.31250000136560452 ) ) ;
#20495=EDGE_CURVE ( 'NONE', #13665, #158, #17057, .T. ) ;
#20498=CARTESIAN_POINT ( 'NONE',  ( 9.920644283265380691E-16, 4.000000000000000000, 9.875000002731196602 ) ) ;
#20501=CARTESIAN_POINT ( 'NONE',  ( 1.025207404391860050E-15, 3.458734125000000326, 11.18750000136560452 ) ) ;
#20502=CARTESIAN_POINT ( 'NONE',  ( 2.828427124746192067, -2.828427124746189847, 14.50000000273119660 ) ) ;
#20503=CARTESIAN_POINT ( 'NONE',  ( 1.025207404391860050E-15, 3.458734125000000770, 10.43750000136560629 ) ) ;
#20513=CARTESIAN_POINT ( 'NONE',  ( 4.000000000000000888, 1.656854249492381248, 14.56250000000001066 ) ) ;
#20521=DIRECTION ( 'NONE',  ( -0.000000000000000000, -0.000000000000000000, -1.000000000000000000 ) ) ;
#20526=CARTESIAN_POINT ( 'NONE',  ( 1.432654583217643163, -3.458734124999999882, 16.00000000136560629 ) ) ;
#20532=VERTEX_POINT ( 'NONE', #13218 ) ;
#20552=CARTESIAN_POINT ( 'NONE',  ( -1.656854249492379250, 4.000000000000000000, 13.93750000273119483 ) ) ;
#20554=CARTESIAN_POINT ( 'NONE',  ( -3.999999999999999112, 0.000000000000000000, 19.56250000136560629 ) ) ;
#20556=CARTESIAN_POINT ( 'NONE',  ( 4.000000000000001776, -1.656854249492379694, 12.56250000273119838 ) ) ;
#20566=CARTESIAN_POINT ( 'NONE',  ( 19.99999999999998934, 4.500000000000003553, -50.00000000000000000 ) ) ;
#20572=ORIENTED_EDGE ( 'NONE', *, *, #21051, .F. ) ;
#20573=VECTOR ( 'NONE', #20575, 1000.000000000000000 ) ;
#20575=DIRECTION ( 'NONE',  ( 0.000000000000000000, -1.000000000000000000, 0.000000000000000000 ) ) ;
#20576=CARTESIAN_POINT ( 'NONE',  ( -1.656854249492380138, -3.999999999999999112, 16.18750000000001066 ) ) ;
#20584=EDGE_CURVE ( 'NONE', #21282, #7575, #12864, .T. ) ;
#20587=CARTESIAN_POINT ( 'NONE',  ( 4.000000000000000888, 4.898587196589412829E-16, 10.62500000273119660 ) ) ;
#20589=CARTESIAN_POINT ( 'NONE',  ( 2.445694354108821411, 2.445694354108820523, 12.06250000136560629 ) ) ;
#20590=DIRECTION ( 'NONE',  ( -1.000000000000000000, 0.000000000000000000, 1.224646799147353207E-16 ) ) ;
#20595=CARTESIAN_POINT ( 'NONE',  ( -3.458734124999998993, 1.432654583217640276, 11.37500000136560452 ) ) ;
#20597=ORIENTED_EDGE ( 'NONE', *, *, #14484, .T. ) ;
#20608=CARTESIAN_POINT ( 'NONE',  ( -2.445694354108819191, 2.445694354108820523, 18.56250000136560629 ) ) ;
#20612=SHAPE_REPRESENTATION ( 'motor', ( #7318 ), #13013 ) ;
#20622=CARTESIAN_POINT ( 'NONE',  ( 1.432654583217641164, 3.458734125000000326, 12.12500000136560629 ) ) ;
#20623=CARTESIAN_POINT ( 'NONE',  ( 4.000000000000000888, 1.656854249492381248, 16.68750000273119838 ) ) ;
#20632=EDGE_CURVE ( 'NONE', #12232, #2705, #20257, .T. ) ;
#20635=CARTESIAN_POINT ( 'NONE',  ( 4.000000000000001776, -1.656854249492379694, 11.43750000000001066 ) ) ;
#20640=ORIENTED_EDGE ( 'NONE', *, *, #9537, .T. ) ;
#20643=CARTESIAN_POINT ( 'NONE',  ( 1.236993788156008760E-15, 0.000000000000000000, 21.31370849898476649 ) ) ;
#20647=CARTESIAN_POINT ( 'NONE',  ( -3.999999999999998224, -1.656854249492383024, 15.06250000000001066 ) ) ;
#20649=CARTESIAN_POINT ( 'NONE',  ( -1.656854249492380138, -3.999999999999999112, 11.18750000000000888 ) ) ;
#20655=CARTESIAN_POINT ( 'NONE',  ( -1.432654583217639832, -3.458734125000000326, 16.87500000136560629 ) ) ;
#20673=CARTESIAN_POINT ( 'NONE',  ( -3.999999999999999112, -1.132742959800665972, 20.04272942837865656 ) ) ;
#20676=CARTESIAN_POINT ( 'NONE',  ( 1.971781867644420635E-15, -4.000000000000000000, 12.37500000273119838 ) ) ;
#20691=CARTESIAN_POINT ( 'NONE',  ( -2.828427124746189403, 2.828427124746190291, 15.00000000273119660 ) ) ;
#20697=CARTESIAN_POINT ( 'NONE',  ( 2.828427124746191179, 2.828427124746190291, 13.62500000000001066 ) ) ;
#20700=CARTESIAN_POINT ( 'NONE',  ( 19.99999999999998934, 7.500000000000001776, -20.00000000000000000 ) ) ;
#20705=PRODUCT_DEFINITION ( 'UNKNOWN', '', #14535, #10049 ) ;
#20708=CARTESIAN_POINT ( 'NONE',  ( 1.432654583217641164, 3.458734125000000326, 14.12500000136560452 ) ) ;
#20726=CARTESIAN_POINT ( 'NONE',  ( -3.458734124999999437, 1.432654583217640498, 18.62500000136560274 ) ) ;
#20733=LINE ( 'NONE', #15392, #2414 ) ;
#20738=CARTESIAN_POINT ( 'NONE',  ( -3.999999999999998224, -1.656854249492383246, 12.18750000273119838 ) ) ;
#20741=FACE_OUTER_BOUND ( 'NONE', #12303, .T. ) ;
#20742=ORIENTED_EDGE ( 'NONE', *, *, #12523, .T. ) ;
#20749=CARTESIAN_POINT ( 'NONE',  ( 1.971781867644420635E-15, -4.000000000000000000, 11.25000000000001066 ) ) ;
#20756=CARTESIAN_POINT ( 'NONE',  ( 3.458734125000002546, -1.432654583217639610, 19.12500000136560629 ) ) ;
#20767=CARTESIAN_POINT ( 'NONE',  ( -2.445694354108819191, 2.445694354108820523, 12.56250000136560629 ) ) ;
#20783=AXIS2_PLACEMENT_3D ( 'NONE', #5690, #23660, #18386 ) ;
#20793=CARTESIAN_POINT ( 'NONE',  ( 2.445694354108821411, 2.445694354108820523, 19.06250000136560629 ) ) ;
#20812=CARTESIAN_POINT ( 'NONE',  ( -1.656854249492379250, 4.000000000000000000, 10.81250000000001243 ) ) ;
#20819=DIRECTION ( 'NONE',  ( 0.000000000000000000, -0.000000000000000000, -1.000000000000000000 ) ) ;
#20821=CARTESIAN_POINT ( 'NONE',  ( -3.458734124999998993, 0.000000000000000000, 13.43750000136560452 ) ) ;
#20832=ORIENTED_EDGE ( 'NONE', *, *, #11992, .F. ) ;
#20836=ORIENTED_EDGE ( 'NONE', *, *, #4539, .T. ) ;
#20840=CARTESIAN_POINT ( 'NONE',  ( 2.445694354108822299, -2.445694354108820079, 17.06250000136560629 ) ) ;
#20852=CARTESIAN_POINT ( 'NONE',  ( 1.656854249492384135, -3.999999999999999112, 10.43750000273119660 ) ) ;
#20855=DIRECTION ( 'NONE',  ( 1.224646799147353207E-16, -0.000000000000000000, 1.000000000000000000 ) ) ;
#20863=CARTESIAN_POINT ( 'NONE',  ( 9.920644283265380691E-16, 4.000000000000000000, 14.75000000000000888 ) ) ;
#20864=CARTESIAN_POINT ( 'NONE',  ( 4.000000000000000888, 4.898587196589412829E-16, 21.31370849898476649 ) ) ;
#20874=DIRECTION ( 'NONE',  ( -0.9413949561959078505, -0.3373062947069097040, 0.000000000000000000 ) ) ;
#20877=CARTESIAN_POINT ( 'NONE',  ( -3.458734124999998993, -1.432654583217642497, 10.75000000136560452 ) ) ;
#20881=DIRECTION ( 'NONE',  ( -1.000000000000000000, 0.000000000000000000, 0.000000000000000000 ) ) ;
#20883=CARTESIAN_POINT ( 'NONE',  ( 1.656854249492384135, -3.999999999999999112, 14.31250000000001066 ) ) ;
#20903=CARTESIAN_POINT ( 'NONE',  ( -2.445694354108819191, 2.445694354108820523, 18.31250000136560274 ) ) ;
#20906=CARTESIAN_POINT ( 'NONE',  ( -20.00000000000001066, 7.500000000000001776, -49.99999999999998579 ) ) ;
#20911=VERTEX_POINT ( 'NONE', #15731 ) ;
#20917=VERTEX_POINT ( 'NONE', #12611 ) ;
#20930=EDGE_CURVE ( 'NONE', #20461, #16525, #12129, .T. ) ;
#20934=CARTESIAN_POINT ( 'NONE',  ( -2.445694354108818303, -2.445694354108820523, 11.56250000136560629 ) ) ;
#20951=ORIENTED_EDGE ( 'NONE', *, *, #10668, .F. ) ;
#20952=CARTESIAN_POINT ( 'NONE',  ( -2.445694354108818303, -2.445694354108820967, 14.81250000136560452 ) ) ;
#20966=CARTESIAN_POINT ( 'NONE',  ( -1.656854249492379250, 4.000000000000000000, 11.93750000273119660 ) ) ;
#20969=CARTESIAN_POINT ( 'NONE',  ( 9.920644283265380691E-16, 4.000000000000000000, 16.87500000273119838 ) ) ;
#20981=ORIENTED_EDGE ( 'NONE', *, *, #11603, .F. ) ;
#20986=AXIS2_PLACEMENT_3D ( 'NONE', #1494, #10163, #19576 ) ;
#20989=CARTESIAN_POINT ( 'NONE',  ( 3.458734125000001658, 1.432654583217640498, 19.25000000136560629 ) ) ;
#20997=CARTESIAN_POINT ( 'NONE',  ( -3.458734124999999437, 0.000000000000000000, 12.68750000136560629 ) ) ;
#21010=DIRECTION ( 'NONE',  ( 1.224646799147353207E-16, -0.000000000000000000, 1.000000000000000000 ) ) ;
#21024=CARTESIAN_POINT ( 'NONE',  ( -3.458734124999998993, 0.000000000000000000, 18.43750000136560629 ) ) ;
#21044=CARTESIAN_POINT ( 'NONE',  ( -3.999999999999999112, 0.000000000000000000, 21.31370849898476649 ) ) ;
#21050=CARTESIAN_POINT ( 'NONE',  ( -3.999999999999999112, 0.000000000000000000, 10.12500000273119660 ) ) ;
#21051=EDGE_CURVE ( 'NONE', #21587, #19809, #22128, .T. ) ;
#21054=CARTESIAN_POINT ( 'NONE',  ( 2.445694354108821411, 2.445694354108820523, 13.06250000136560452 ) ) ;
#21065=CARTESIAN_POINT ( 'NONE',  ( -3.999999999999999112, 1.656854249492380582, 16.06250000273119838 ) ) ;
#21066=ORIENTED_EDGE ( 'NONE', *, *, #1176, .F. ) ;
#21075=VERTEX_POINT ( 'NONE', #16415 ) ;
#21076=CARTESIAN_POINT ( 'NONE',  ( -3.458734124999998993, -1.432654583217642497, 11.75000000136560629 ) ) ;
#21083=FACE_BOUND ( 'NONE', #3046, .T. ) ;
#21087=CARTESIAN_POINT ( 'NONE',  ( 4.000000000000001776, -1.656854249492379694, 13.56250000273119660 ) ) ;
#21089=ORIENTED_EDGE ( 'NONE', *, *, #21361, .F. ) ;
#21090=DIRECTION ( 'NONE',  ( 1.000000000000000000, 0.000000000000000000, 0.000000000000000000 ) ) ;
#21093=ADVANCED_FACE ( 'NONE', ( #9467 ), #10923, .T. ) ;
#21094=EDGE_CURVE ( 'NONE', #13926, #12919, #12837, .T. ) ;
#21098=ADVANCED_FACE ( 'NONE', ( #21894 ), #18202, .F. ) ;
#21105=CARTESIAN_POINT ( 'NONE',  ( -3.458734124999999437, 1.432654583217640498, 19.62500000136560629 ) ) ;
#21106=CARTESIAN_POINT ( 'NONE',  ( 4.000000000000000888, 4.898587196589412829E-16, 14.62500000273119660 ) ) ;
#21114=VECTOR ( 'NONE', #21311, 1000.000000000000000 ) ;
#21119=VERTEX_POINT ( 'NONE', #7328 ) ;
#21130=SURFACE_SIDE_STYLE ('',( #12428 ) ) ;
#21139=CARTESIAN_POINT ( 'NONE',  ( 1.432654583217641164, 3.458734125000000326, 17.12500000136560629 ) ) ;
#21154=CARTESIAN_POINT ( 'NONE',  ( -3.999999999999999112, 1.656854249492380582, 17.93750000000001421 ) ) ;
#21166=CARTESIAN_POINT ( 'NONE',  ( -3.458734124999998993, 0.000000000000000000, 11.43750000136560452 ) ) ;
#21168=DIRECTION ( 'NONE',  ( 1.000000000000000000, 0.000000000000000000, 0.000000000000000000 ) ) ;
#21171=CARTESIAN_POINT ( 'NONE',  ( 4.000000000000000888, 4.898587196589412829E-16, 15.50000000000001066 ) ) ;
#21175=CARTESIAN_POINT ( 'NONE',  ( 1.971781867644420635E-15, -4.000000000000000000, 13.37500000273119660 ) ) ;
#21178=ORIENTED_EDGE ( 'NONE', *, *, #10668, .T. ) ;
#21182=CARTESIAN_POINT ( 'NONE',  ( 1.432654583217643163, -3.458734124999999882, 13.00000000136560629 ) ) ;
#21183=DIRECTION ( 'NONE',  ( -0.000000000000000000, -1.000000000000000000, 0.000000000000000000 ) ) ;
#21187=DIRECTION ( 'NONE',  ( 0.000000000000000000, -1.000000000000000000, 0.000000000000000000 ) ) ;
#21197=CARTESIAN_POINT ( 'NONE',  ( -3.999999999999998224, -1.656854249492383024, 13.06250000000001243 ) ) ;
#21199=CARTESIAN_POINT ( 'NONE',  ( 4.000000000000001776, -1.656854249492379694, 11.56250000273119838 ) ) ;
#21219=CARTESIAN_POINT ( 'NONE',  ( 1.025207404391860050E-15, 3.458734125000000770, 15.43750000136560452 ) ) ;
#21220=CARTESIAN_POINT ( 'NONE',  ( -3.999999999999998224, -1.656854249492383246, 14.18750000273119483 ) ) ;
#21236=CARTESIAN_POINT ( 'NONE',  ( -2.828427124746188515, -2.828427124746190735, 15.25000000273119660 ) ) ;
#21248=EDGE_CURVE ( 'NONE', #13749, #3286, #2489, .T. ) ;
#21253=CARTESIAN_POINT ( 'NONE',  ( 1.872352939448454495E-15, -3.458734125000000326, 14.68750000136560452 ) ) ;
#21271=CARTESIAN_POINT ( 'NONE',  ( 14.99999999999995737, -15.00000000000000000, -50.00000000000000000 ) ) ;
#21278=CARTESIAN_POINT ( 'NONE',  ( -3.458734124999998993, -1.432654583217642497, 10.50000000136560452 ) ) ;
#21282=VERTEX_POINT ( 'NONE', #8027 ) ;
#21287=ORIENTED_EDGE ( 'NONE', *, *, #10860, .F. ) ;
#21289=CARTESIAN_POINT ( 'NONE',  ( -3.999999999999998224, -1.656854249492383024, 13.18750000273119660 ) ) ;
#21292=ORIENTED_EDGE ( 'NONE', *, *, #21248, .T. ) ;
#21296=ORIENTED_EDGE ( 'NONE', *, *, #12756, .T. ) ;
#21297=CARTESIAN_POINT ( 'NONE',  ( 2.445694354108822299, -2.445694354108820079, 12.06250000136560629 ) ) ;
#21298=ADVANCED_FACE ( 'NONE', ( #694 ), #927, .T. ) ;
#21303=FACE_OUTER_BOUND ( 'NONE', #2679, .T. ) ;
#21311=DIRECTION ( 'NONE',  ( -1.000000000000000000, 0.000000000000000000, 1.982541115402065110E-16 ) ) ;
#21312=CARTESIAN_POINT ( 'NONE',  ( 2.445694354108821411, 2.445694354108820523, 19.06250000136560629 ) ) ;
#21329=CARTESIAN_POINT ( 'NONE',  ( 2.828427124746191179, 2.828427124746190291, 19.62500000000001066 ) ) ;
#21338=VECTOR ( 'NONE', #17004, 1000.000000000000000 ) ;
#21339=CARTESIAN_POINT ( 'NONE',  ( 3.458734125000001658, 4.235727675282972223E-16, 15.18750000136560452 ) ) ;
#21345=CARTESIAN_POINT ( 'NONE',  ( 1.971781867644420635E-15, -4.000000000000000000, 18.37500000273119483 ) ) ;
#21348=AXIS2_PLACEMENT_3D ( 'NONE', #10138, #996, #2439 ) ;
#21359=CARTESIAN_POINT ( 'NONE',  ( 34.99999999999999289, 4.500000000000001776, -50.00000000000000000 ) ) ;
#21361=EDGE_CURVE ( 'NONE', #16525, #17599, #3004, .T. ) ;
#21362=FILL_AREA_STYLE_COLOUR ( '', #11483 ) ;
#21376=CARTESIAN_POINT ( 'NONE',  ( 3.458734125000001214, 4.235727675282971730E-16, 12.93750000136560452 ) ) ;
#21379=DIRECTION ( 'NONE',  ( -0.000000000000000000, -0.000000000000000000, -1.000000000000000000 ) ) ;
#21385=EDGE_LOOP ( 'NONE', ( #17958, #18647, #2811, #7329 ) ) ;
#21399=LINE ( 'NONE', #22979, #6496 ) ;
#21406=CARTESIAN_POINT ( 'NONE',  ( 1.432654583217643163, -3.458734124999999882, 19.00000000136560629 ) ) ;
#21425=CARTESIAN_POINT ( 'NONE',  ( 2.445694354108821411, 2.445694354108820523, 13.31250000136560452 ) ) ;
#21437=CARTESIAN_POINT ( 'NONE',  ( -1.432654583217639610, -3.458734124999999882, 15.62500000136560629 ) ) ;
#21440=ORIENTED_EDGE ( 'NONE', *, *, #10831, .F. ) ;
#21458=CARTESIAN_POINT ( 'NONE',  ( 1.432654583217641386, 3.458734125000000770, 17.37500000136560985 ) ) ;
#21482=CARTESIAN_POINT ( 'NONE',  ( -3.999999999999999112, 0.000000000000000000, 11.00000000000001066 ) ) ;
#21485=EDGE_CURVE ( 'NONE', #839, #21889, #21801, .T. ) ;
#21495=CARTESIAN_POINT ( 'NONE',  ( 3.458734125000001214, 1.432654583217640498, 14.00000000136560452 ) ) ;
#21500=ORIENTED_EDGE ( 'NONE', *, *, #396, .F. ) ;
#21509=CARTESIAN_POINT ( 'NONE',  ( 14.99999999999999645, -10.00000000000000000, -20.00000000000000355 ) ) ;
#21523=FACE_OUTER_BOUND ( 'NONE', #15832, .T. ) ;
#21524=CARTESIAN_POINT ( 'NONE',  ( -2.445694354108818303, -2.445694354108820967, 18.81250000136560629 ) ) ;
#21532=CARTESIAN_POINT ( 'NONE',  ( -1.656854249492379472, 4.000000000000000000, 10.93750000273119660 ) ) ;
#21543=CARTESIAN_POINT ( 'NONE',  ( -3.999999999999999112, 0.000000000000000000, 20.00000000000001066 ) ) ;
#21555=CARTESIAN_POINT ( 'NONE',  ( 1.872352939448454495E-15, -3.458734125000000326, 17.68750000136560274 ) ) ;
#21565=CYLINDRICAL_SURFACE ( 'NONE', #14857, 4.000000000000000000 ) ;
#21575=CARTESIAN_POINT ( 'NONE',  ( 3.458734125000002546, -1.432654583217639610, 16.12500000136560629 ) ) ;
#21581=CARTESIAN_POINT ( 'NONE',  ( -2.828427124746189403, 2.828427124746190291, 19.00000000273119838 ) ) ;
#21587=VERTEX_POINT ( 'NONE', #7411 ) ;
#21595=CARTESIAN_POINT ( 'NONE',  ( 1.656854249492384135, -3.999999999999999112, 15.31250000000000888 ) ) ;
#21597=EDGE_CURVE ( 'NONE', #17601, #21119, #1465, .T. ) ;
#21603=VERTEX_POINT ( 'NONE', #10785 ) ;
#21609=DIRECTION ( 'NONE',  ( -0.000000000000000000, -0.000000000000000000, -1.000000000000000000 ) ) ;
#21614=CARTESIAN_POINT ( 'NONE',  ( -3.458734124999998105, 1.432654583217640276, 14.37500000136560452 ) ) ;
#21662=CARTESIAN_POINT ( 'NONE',  ( 9.920644283265380691E-16, 4.000000000000000000, 18.75000000000001066 ) ) ;
#21663=CARTESIAN_POINT ( 'NONE',  ( 2.828427124746192067, -2.828427124746189847, 17.37500000000001066 ) ) ;
#21678=CARTESIAN_POINT ( 'NONE',  ( -3.458734124999998993, -1.432654583217642497, 16.50000000136560629 ) ) ;
#21699=CARTESIAN_POINT ( 'NONE',  ( 3.458734125000002546, -1.432654583217639610, 17.12500000136560629 ) ) ;
#21700=CARTESIAN_POINT ( 'NONE',  ( -2.828427124746188515, -2.828427124746190735, 10.25000000273119660 ) ) ;
#21703=AXIS2_PLACEMENT_3D ( 'NONE', #3057, #12311, #19574 ) ;
#21707=CARTESIAN_POINT ( 'NONE',  ( 1.656854249492381470, 4.000000000000000000, 18.81250000273119838 ) ) ;
#21716=CARTESIAN_POINT ( 'NONE',  ( -2.828427124746189403, 2.828427124746190291, 16.87500000000001066 ) ) ;
#21724=FACE_OUTER_BOUND ( 'NONE', #13365, .T. ) ;
#21735=CARTESIAN_POINT ( 'NONE',  ( -3.458734124999998105, -1.432654583217642275, 10.50000000136560452 ) ) ;
#21738=ORIENTED_EDGE ( 'NONE', *, *, #17970, .F. ) ;
#21746=VECTOR ( 'NONE', #17834, 1000.000000000000000 ) ;
#21759=ORIENTED_EDGE ( 'NONE', *, *, #14442, .F. ) ;
#21760=CARTESIAN_POINT ( 'NONE',  ( 4.000000000000000888, 1.656854249492381248, 18.68750000273119483 ) ) ;
#21786=CARTESIAN_POINT ( 'NONE',  ( 1.656854249492381470, 4.000000000000000000, 18.68750000000001066 ) ) ;
#21787=CARTESIAN_POINT ( 'NONE',  ( -1.656854249492380138, -3.999999999999999112, 18.18750000000001066 ) ) ;
#21799=CARTESIAN_POINT ( 'NONE',  ( 3.458734125000002102, -1.432654583217639610, 17.87500000136560274 ) ) ;
#21801=( BOUNDED_CURVE ( )  B_SPLINE_CURVE ( 2, ( #5712, #9091, #18172, #14966, #21868, #5473, #194, #14839, #23564 ),
 .UNSPECIFIED., .F., .F. ) 
 B_SPLINE_CURVE_WITH_KNOTS ( ( 3, 2, 2, 2, 3 ),
 ( 0.1499999999999999944, 0.1625000000000000056, 0.1749999999999999889, 0.1875000000000000000, 0.2000000000000000111 ),
 .UNSPECIFIED. ) 
 CURVE ( )  GEOMETRIC_REPRESENTATION_ITEM ( )  RATIONAL_B_SPLINE_CURVE ( ( 1.000000000000000000, 0.9238795325112867385, 1.000000000000000000, 0.9238795325112867385, 1.000000000000000000, 0.9238795325112867385, 1.000000000000000000, 0.9238795325112867385, 1.000000000000000000 ) ) 
 REPRESENTATION_ITEM ( '' )  );
#21805=CARTESIAN_POINT ( 'NONE',  ( 3.458734125000001214, 1.432654583217640498, 16.00000000136560629 ) ) ;
#21818=AXIS2_PLACEMENT_3D ( 'NONE', #7072, #6713, #3344 ) ;
#21824=CARTESIAN_POINT ( 'NONE',  ( 1.432654583217643163, -3.458734124999999882, 11.00000000136560452 ) ) ;
#21825=CARTESIAN_POINT ( 'NONE',  ( 2.828427124746191179, 2.828427124746190291, 11.75000000273119660 ) ) ;
#21834=EDGE_CURVE ( 'NONE', #22990, #4495, #17581, .T. ) ;
#21843=CARTESIAN_POINT ( 'NONE',  ( -2.828427124746189403, 2.828427124746190291, 18.87500000000001066 ) ) ;
#21847=DIRECTION ( 'NONE',  ( -1.224646799147353207E-16, 0.000000000000000000, -1.000000000000000000 ) ) ;
#21859=CARTESIAN_POINT ( 'NONE',  ( 4.000000000000000888, 4.898587196589412829E-16, 11.62500000273119660 ) ) ;
#21861=LINE ( 'NONE', #8975, #23116 ) ;
#21868=CARTESIAN_POINT ( 'NONE',  ( 1.971781867644420635E-15, -4.000000000000000000, 18.25000000000001066 ) ) ;
#21877=CARTESIAN_POINT ( 'NONE',  ( 4.000000000000001776, -1.656854249492379694, 16.56250000273119838 ) ) ;
#21887=CARTESIAN_POINT ( 'NONE',  ( -20.00000000000001066, 9.999999999999964473, -49.99999999999999289 ) ) ;
#21889=VERTEX_POINT ( 'NONE', #15670 ) ;
#21894=FACE_OUTER_BOUND ( 'NONE', #7758, .T. ) ;
#21895=ORIENTED_EDGE ( 'NONE', *, *, #21930, .F. ) ;
#21896=ADVANCED_FACE ( 'NONE', ( #1136 ), #17913, .T. ) ;
#21898=CARTESIAN_POINT ( 'NONE',  ( -2.828427124746189403, 2.828427124746190291, 16.87500000000001066 ) ) ;
#21899=CARTESIAN_POINT ( 'NONE',  ( 27.50000000000000000, 7.500000000000001776, -36.31025403784445871 ) ) ;
#21907=CARTESIAN_POINT ( 'NONE',  ( 1.432654583217641164, 3.458734125000000326, 16.12500000136560629 ) ) ;
#21911=CARTESIAN_POINT ( 'NONE',  ( -1.432654583217639610, -3.458734124999999882, 13.62500000136560452 ) ) ;
#21913=ORIENTED_EDGE ( 'NONE', *, *, #7439, .T. ) ;
#21921=VECTOR ( 'NONE', #20521, 1000.000000000000000 ) ;
#21923=ADVANCED_FACE ( 'NONE', ( #23295 ), #6670, .F. ) ;
#21929=MANIFOLD_SOLID_BREP ( 'M5 Clearance Hole1', #20396 ) ;
#21930=EDGE_CURVE ( 'NONE', #4420, #16525, #3757, .T. ) ;
#21933=CARTESIAN_POINT ( 'NONE',  ( 3.458734125000001658, 4.235727675282972223E-16, 11.18750000136560452 ) ) ;
#21936=LINE ( 'NONE', #16689, #17730 ) ;
#21938=CARTESIAN_POINT ( 'NONE',  ( -1.656854249492380138, -3.999999999999999112, 16.31250000273119483 ) ) ;
#21939=CARTESIAN_POINT ( 'NONE',  ( -3.458734124999998993, 0.000000000000000000, 19.56250000136560629 ) ) ;
#21948=CARTESIAN_POINT ( 'NONE',  ( 4.000000000000000888, 1.656854249492381248, 17.56250000000001421 ) ) ;
#21963=VECTOR ( 'NONE', #7661, 1000.000000000000000 ) ;
#21965=CARTESIAN_POINT ( 'NONE',  ( -2.445694354108819191, 2.445694354108820523, 19.56250000136560629 ) ) ;
#21982=VECTOR ( 'NONE', #6336, 1000.000000000000000 ) ;
#21990=CARTESIAN_POINT ( 'NONE',  ( 1.656854249492384135, -3.999999999999999112, 16.43750000273119838 ) ) ;
#21995=CARTESIAN_POINT ( 'NONE',  ( 27.50000000000000000, 7.500000000000002665, -31.01025403784447576 ) ) ;
#22004=VERTEX_POINT ( 'NONE', #7388 ) ;
#22010=CARTESIAN_POINT ( 'NONE',  ( -2.828427124746189403, 2.828427124746190291, 19.00000000273119838 ) ) ;
#22011=CARTESIAN_POINT ( 'NONE',  ( 4.000000000000001776, -1.656854249492379694, 18.43750000000000711 ) ) ;
#22020=CARTESIAN_POINT ( 'NONE',  ( -3.458734124999998993, 0.000000000000000000, 18.43750000136560629 ) ) ;
#22025=CARTESIAN_POINT ( 'NONE',  ( -3.458734124999998993, -1.432654583217642497, 14.50000000136560629 ) ) ;
#22033=CARTESIAN_POINT ( 'NONE',  ( -2.828427124746188515, -2.828427124746190735, 17.12500000000001066 ) ) ;
#22036=CARTESIAN_POINT ( 'NONE',  ( 2.445694354108822299, -2.445694354108820079, 19.06250000136560629 ) ) ;
#22041=CARTESIAN_POINT ( 'NONE',  ( 2.445694354108822299, -2.445694354108820079, 13.06250000136560629 ) ) ;
#22048=CARTESIAN_POINT ( 'NONE',  ( 1.656854249492381470, 4.000000000000000000, 15.81250000273119660 ) ) ;
#22051=ORIENTED_EDGE ( 'NONE', *, *, #19552, .F. ) ;
#22054=EDGE_LOOP ( 'NONE', ( #14927, #6096, #16242, #5823, #13743, #8282, #23350, #13802, #18870, #8042, #13657, #8126, #5941, #13107, #16605, #1776, #1166, #22051, #23573, #15041, #9917, #6190, #21738, #19773 ) ) ;
#22057=ADVANCED_FACE ( 'NONE', ( #14456, #5212 ), #12678, .T. ) ;
#22060=CARTESIAN_POINT ( 'NONE',  ( 4.000000000000000888, 1.656854249492381248, 18.56250000000001421 ) ) ;
#22077=CARTESIAN_POINT ( 'NONE',  ( 1.432654583217641386, 3.458734125000000770, 14.37500000136560452 ) ) ;
#22089=EDGE_CURVE ( 'NONE', #21603, #1132, #3367, .T. ) ;
#22092=PLANE ( 'NONE',  #4878 ) ;
#22103=CARTESIAN_POINT ( 'NONE',  ( -3.999999999999999112, 0.000000000000000000, 19.12500000273119838 ) ) ;
#22106=AXIS2_PLACEMENT_3D ( 'NONE', #12730, #11161, #23591 ) ;
#22112=DIRECTION ( 'NONE',  ( -1.224646799147353207E-16, 0.000000000000000000, -1.000000000000000000 ) ) ;
#22113=VERTEX_POINT ( 'NONE', #23484 ) ;
#22114=DIRECTION ( 'NONE',  ( 0.000000000000000000, -0.000000000000000000, -1.000000000000000000 ) ) ;
#22118=VECTOR ( 'NONE', #709, 1000.000000000000000 ) ;
#22128=LINE ( 'NONE', #5391, #22521 ) ;
#22131=CARTESIAN_POINT ( 'NONE',  ( 2.828427124746191179, 2.828427124746190291, 18.75000000273119483 ) ) ;
#22133=CARTESIAN_POINT ( 'NONE',  ( 1.971781867644420635E-15, -4.000000000000000000, 14.25000000000001066 ) ) ;
#22144=CARTESIAN_POINT ( 'NONE',  ( -1.432654583217639610, -3.458734124999999882, 15.62500000136560629 ) ) ;
#22150=CARTESIAN_POINT ( 'NONE',  ( -1.432654583217638944, 3.458734125000000326, 12.25000000136560452 ) ) ;
#22159=CARTESIAN_POINT ( 'NONE',  ( 2.828427124746192067, -2.828427124746189847, 17.37500000000001066 ) ) ;
#22163=CARTESIAN_POINT ( 'NONE',  ( 3.458734125000001658, 4.235727675282972223E-16, 18.18750000136560274 ) ) ;
#22171=CARTESIAN_POINT ( 'NONE',  ( 1.432654583217641386, 3.458734125000000770, 11.37500000136560452 ) ) ;
#22172=CARTESIAN_POINT ( 'NONE',  ( -20.00000000000001066, 4.500000000000003553, -49.99999999999999289 ) ) ;
#22177=CARTESIAN_POINT ( 'NONE',  ( -2.828427124746188515, -2.828427124746190735, 16.25000000273119838 ) ) ;
#22189=CARTESIAN_POINT ( 'NONE',  ( -3.999999999999998224, -1.656854249492383246, 13.06250000000001066 ) ) ;
#22193=EDGE_CURVE ( 'NONE', #19809, #13130, #12049, .T. ) ;
#22204=CARTESIAN_POINT ( 'NONE',  ( 3.458734125000001658, 1.432654583217640498, 13.25000000136560452 ) ) ;
#22214=ORIENTED_EDGE ( 'NONE', *, *, #5730, .F. ) ;
#22230=CARTESIAN_POINT ( 'NONE',  ( -3.999999999999999112, 0.000000000000000000, 15.12500000273119660 ) ) ;
#22238=CARTESIAN_POINT ( 'NONE',  ( -20.00000000000001066, 9.999999999999964473, -49.99999999999999289 ) ) ;
#22249=DIRECTION ( 'NONE',  ( -0.000000000000000000, 1.000000000000000000, -0.000000000000000000 ) ) ;
#22253=CARTESIAN_POINT ( 'NONE',  ( 4.000000000000000888, 1.656854249492381248, 14.56250000000001066 ) ) ;
#22266=CARTESIAN_POINT ( 'NONE',  ( 2.445694354108821411, 2.445694354108820523, 17.06250000136560629 ) ) ;
#22271=CARTESIAN_POINT ( 'NONE',  ( 3.458734125000001214, 1.432654583217640498, 15.00000000136560629 ) ) ;
#22281=VERTEX_POINT ( 'NONE', #23310 ) ;
#22282=CARTESIAN_POINT ( 'NONE',  ( 1.872352939448454495E-15, -3.458734125000000770, 16.93750000136560629 ) ) ;
#22290=CARTESIAN_POINT ( 'NONE',  ( 1.025207404391860050E-15, 3.458734125000000770, 11.43750000136560452 ) ) ;
#22295=CARTESIAN_POINT ( 'NONE',  ( 2.445694354108821411, 2.445694354108820523, 12.06250000136560629 ) ) ;
#22296=CARTESIAN_POINT ( 'NONE',  ( 1.656854249492381470, 4.000000000000000000, 16.81250000273119838 ) ) ;
#22308=CARTESIAN_POINT ( 'NONE',  ( 1.656854249492381470, 4.000000000000000000, 11.68750000000001066 ) ) ;
#22310=CARTESIAN_POINT ( 'NONE',  ( 2.828427124746191179, 2.828427124746190291, 14.62500000000000888 ) ) ;
#22315=B_SPLINE_CURVE_WITH_KNOTS ( 'NONE', 1,
 ( #15040, #20503 ),
 .UNSPECIFIED., .F., .F.,
 ( 2, 2 ),
 ( 0.000000000000000000, 1.000000000000000000 ),
 .UNSPECIFIED. ) ;
#22317=CARTESIAN_POINT ( 'NONE',  ( 4.000000000000000888, 4.898587196589412829E-16, 21.31370849898476649 ) ) ;
#22321=CARTESIAN_POINT ( 'NONE',  ( -3.458734124999998993, -1.432654583217642497, 16.75000000136560629 ) ) ;
#22322=FACE_OUTER_BOUND ( 'NONE', #6125, .T. ) ;
#22328=CARTESIAN_POINT ( 'NONE',  ( 2.828427124746192067, -2.828427124746189847, 14.37500000000001066 ) ) ;
#22333=DIRECTION ( 'NONE',  ( -1.224646799147353207E-16, 0.000000000000000000, -1.000000000000000000 ) ) ;
#22336=ORIENTED_EDGE ( 'NONE', *, *, #10831, .T. ) ;
#22346=CARTESIAN_POINT ( 'NONE',  ( -3.999999999999999112, 0.000000000000000000, 13.12500000273119660 ) ) ;
#22349=PLANE ( 'NONE',  #12314 ) ;
#22365=ADVANCED_FACE ( 'NONE', ( #22322 ), #17078, .F. ) ;
#22371=CARTESIAN_POINT ( 'NONE',  ( 1.656854249492381470, 4.000000000000000000, 13.68750000000001066 ) ) ;
#22375=CARTESIAN_POINT ( 'NONE',  ( -2.828427124746189403, 2.828427124746190291, 18.00000000273119483 ) ) ;
#22382=CARTESIAN_POINT ( 'NONE',  ( 34.99999999999999289, 4.500000000000001776, -50.00000000000000000 ) ) ;
#22384=CARTESIAN_POINT ( 'NONE',  ( -2.445694354108819191, 2.445694354108820523, 13.31250000136560452 ) ) ;
#22390=CARTESIAN_POINT ( 'NONE',  ( 3.458734125000002102, -1.432654583217639610, 13.87500000136560452 ) ) ;
#22406=CARTESIAN_POINT ( 'NONE',  ( -3.458734124999999437, 1.432654583217640498, 16.62500000136560629 ) ) ;
#22415=CARTESIAN_POINT ( 'NONE',  ( -2.445694354108819191, 2.445694354108820523, 11.31250000136560452 ) ) ;
#22416=CARTESIAN_POINT ( 'NONE',  ( -3.999999999999998224, -1.656854249492383246, 14.18750000273119483 ) ) ;
#22426=CARTESIAN_POINT ( 'NONE',  ( 2.828427124746191179, 2.828427124746190291, 13.62500000000001066 ) ) ;
#22429=DIRECTION ( 'NONE',  ( 1.224646799147353207E-16, -0.000000000000000000, 1.000000000000000000 ) ) ;
#22441=CARTESIAN_POINT ( 'NONE',  ( 2.445694354108821411, 2.445694354108820523, 15.31250000136560452 ) ) ;
#22461=CARTESIAN_POINT ( 'NONE',  ( 4.000000000000001776, -1.656854249492379694, 19.43750000000001066 ) ) ;
#22465=CARTESIAN_POINT ( 'NONE',  ( -3.999999999999999112, 1.656854249492380804, 12.06250000273119838 ) ) ;
#22470=CARTESIAN_POINT ( 'NONE',  ( -1.432654583217639610, -3.458734124999999882, 17.62500000136560274 ) ) ;
#22490=CARTESIAN_POINT ( 'NONE',  ( 1.656854249492384135, -3.999999999999999112, 15.31250000000000888 ) ) ;
#22498=CARTESIAN_POINT ( 'NONE',  ( -3.999999999999999112, 0.000000000000000000, 18.12500000273119483 ) ) ;
#22506=CARTESIAN_POINT ( 'NONE',  ( 3.458734125000001214, 1.432654583217640498, 15.00000000136560629 ) ) ;
#22512=CARTESIAN_POINT ( 'NONE',  ( -2.445694354108819191, 2.445694354108820523, 11.31250000136560452 ) ) ;
#22521=VECTOR ( 'NONE', #3824, 1000.000000000000000 ) ;
#22525=AXIS2_PLACEMENT_3D ( 'NONE', #3460, #16050, #19734 ) ;
#22528=CARTESIAN_POINT ( 'NONE',  ( 1.432654583217641386, 3.458734125000000770, 16.37500000136560629 ) ) ;
#22544=CARTESIAN_POINT ( 'NONE',  ( 2.445694354108821411, 2.445694354108820523, 11.06250000136560452 ) ) ;
#22545=CARTESIAN_POINT ( 'NONE',  ( 4.000000000000000888, 1.656854249492381248, 12.68750000273119660 ) ) ;
#22557=CARTESIAN_POINT ( 'NONE',  ( 2.828427124746191179, 2.828427124746190291, 14.62500000000000888 ) ) ;
#22573=EDGE_CURVE ( 'NONE', #15974, #22990, #7251, .T. ) ;
#22578=CARTESIAN_POINT ( 'NONE',  ( 1.872352939448454495E-15, -3.458734125000000770, 14.93750000136560452 ) ) ;
#22602=CARTESIAN_POINT ( 'NONE',  ( -1.432654583217639610, -3.458734124999999882, 18.62500000136560629 ) ) ;
#22619=CARTESIAN_POINT ( 'NONE',  ( 2.828427124746192067, -2.828427124746189847, 15.37500000000001066 ) ) ;
#22628=FACE_BOUND ( 'NONE', #277, .T. ) ;
#22630=CARTESIAN_POINT ( 'NONE',  ( 1.432654583217643163, -3.458734124999999437, 11.75000000136560629 ) ) ;
#22636=CARTESIAN_POINT ( 'NONE',  ( 3.458734125000002102, -1.432654583217639610, 10.87500000136560452 ) ) ;
#22647=CARTESIAN_POINT ( 'NONE',  ( 2.445694354108821411, 2.445694354108820523, 16.31250000136560629 ) ) ;
#22658=CARTESIAN_POINT ( 'NONE',  ( 4.000000000000001776, -1.656854249492379694, 10.56250000273119660 ) ) ;
#22660=ORIENTED_EDGE ( 'NONE', *, *, #9397, .F. ) ;
#22661=EDGE_CURVE ( 'NONE', #19691, #16922, #1826, .T. ) ;
#22669=CARTESIAN_POINT ( 'NONE',  ( -3.999999999999998224, -1.656854249492383246, 15.06250000000001066 ) ) ;
#22686=CARTESIAN_POINT ( 'NONE',  ( 1.432654583217641386, 3.458734125000000770, 12.37500000136560629 ) ) ;
#22714=CARTESIAN_POINT ( 'NONE',  ( 3.458734125000002102, -1.432654583217639610, 18.87500000136560629 ) ) ;
#22727=EDGE_CURVE ( 'NONE', #7848, #7815, #11082, .T. ) ;
#22733=CARTESIAN_POINT ( 'NONE',  ( -3.999999999999999112, 0.000000000000000000, 18.00000000000001066 ) ) ;
#22737=CARTESIAN_POINT ( 'NONE',  ( -2.828427124746188515, -2.828427124746190735, 19.12500000000001066 ) ) ;
#22742=CARTESIAN_POINT ( 'NONE',  ( -3.999999999999999112, 0.000000000000000000, 19.00000000000001066 ) ) ;
#22744=CARTESIAN_POINT ( 'NONE',  ( -1.432654583217638944, 3.458734125000000326, 13.25000000136560452 ) ) ;
#22752=CARTESIAN_POINT ( 'NONE',  ( 3.458734125000001214, 1.432654583217640498, 11.00000000136560452 ) ) ;
#22763=CARTESIAN_POINT ( 'NONE',  ( 1.872352939448454495E-15, -3.458734125000000770, 12.93750000136560629 ) ) ;
#22768=EDGE_CURVE ( 'NONE', #5706, #14730, #14937, .T. ) ;
#22775=CARTESIAN_POINT ( 'NONE',  ( -3.999999999999999112, 0.000000000000000000, 11.12500000273119660 ) ) ;
#22796=FACE_OUTER_BOUND ( 'NONE', #2225, .T. ) ;
#22804=CARTESIAN_POINT ( 'NONE',  ( 1.025207404391860050E-15, 3.458734125000000770, 11.43750000136560452 ) ) ;
#22830=CARTESIAN_POINT ( 'NONE',  ( 2.445694354108821855, -2.445694354108820079, 18.81250000136560629 ) ) ;
#22842=CARTESIAN_POINT ( 'NONE',  ( 1.236993788156008760E-15, 0.000000000000000000, 21.31370849898476649 ) ) ;
#22846=ORIENTED_EDGE ( 'NONE', *, *, #16827, .T. ) ;
#22862=CARTESIAN_POINT ( 'NONE',  ( 3.458734125000001214, 4.235727675282971730E-16, 12.93750000136560452 ) ) ;
#22864=EDGE_CURVE ( 'NONE', #14597, #10607, #22315, .T. ) ;
#22873=CARTESIAN_POINT ( 'NONE',  ( 27.50000000000000000, 7.500000000000002665, -33.66025403784446723 ) ) ;
#22884=CARTESIAN_POINT ( 'NONE',  ( -2.445694354108818303, -2.445694354108820967, 11.81250000136560629 ) ) ;
#22897=CARTESIAN_POINT ( 'NONE',  ( -3.999999999999999112, 0.000000000000000000, 12.12500000273119838 ) ) ;
#22911=CARTESIAN_POINT ( 'NONE',  ( 1.656854249492381470, 4.000000000000000000, 19.68750000000001066 ) ) ;
#22920=CARTESIAN_POINT ( 'NONE',  ( -3.999999999999998224, -1.656854249492383246, 15.18750000273119660 ) ) ;
#22935=CARTESIAN_POINT ( 'NONE',  ( 4.000000000000001776, -1.656854249492379694, 15.56250000273119660 ) ) ;
#22957=CARTESIAN_POINT ( 'NONE',  ( 1.432654583217641164, 3.458734125000000326, 18.12500000136560274 ) ) ;
#22962=CARTESIAN_POINT ( 'NONE',  ( -3.999999999999999112, 0.000000000000000000, 12.00000000000001066 ) ) ;
#22979=CARTESIAN_POINT ( 'NONE',  ( 9.920644283265380691E-16, 4.000000000000000000, 21.31370849898476649 ) ) ;
#22983=VECTOR ( 'NONE', #19860, 1000.000000000000114 ) ;
#22987=CARTESIAN_POINT ( 'NONE',  ( -1.432654583217638944, 3.458734125000000326, 10.25000000136560452 ) ) ;
#22990=VERTEX_POINT ( 'NONE', #8437 ) ;
#22992=CARTESIAN_POINT ( 'NONE',  ( -2.828427124746189403, 2.828427124746190291, 15.87500000000001066 ) ) ;
#22996=CARTESIAN_POINT ( 'NONE',  ( 4.000000000000001776, -1.656854249492379694, 13.56250000273119660 ) ) ;
#23006=CARTESIAN_POINT ( 'NONE',  ( 1.872352939448454495E-15, -3.458734125000000770, 13.93750000136560629 ) ) ;
#23016=CARTESIAN_POINT ( 'NONE',  ( -3.999999999999999112, 0.000000000000000000, 21.31370849898476649 ) ) ;
#23018=CARTESIAN_POINT ( 'NONE',  ( -2.828427124746188515, -2.828427124746190735, 11.25000000273119660 ) ) ;
#23021=CARTESIAN_POINT ( 'NONE',  ( 4.000000000000000888, 4.898587196589412829E-16, 16.62500000273119838 ) ) ;
#23022=ORIENTED_EDGE ( 'NONE', *, *, #11603, .T. ) ;
#23036=CARTESIAN_POINT ( 'NONE',  ( 1.025207404391860050E-15, 3.458734125000000326, 10.18750000136560629 ) ) ;
#23037=CARTESIAN_POINT ( 'NONE',  ( -1.656854249492380138, -3.999999999999999112, 14.31250000273119660 ) ) ;
#23043=CARTESIAN_POINT ( 'NONE',  ( -1.432654583217639832, -3.458734125000000326, 10.87500000136560452 ) ) ;
#23047=LINE ( 'NONE', #9053, #12019 ) ;
#23062=CARTESIAN_POINT ( 'NONE',  ( -1.656854249492380138, -3.999999999999999112, 17.31250000273119483 ) ) ;
#23063=ADVANCED_FACE ( 'NONE', ( #860 ), #9878, .F. ) ;
#23067=CARTESIAN_POINT ( 'NONE',  ( 1.432654583217643163, -3.458734124999999437, 14.75000000136560452 ) ) ;
#23075=ORIENTED_EDGE ( 'NONE', *, *, #4507, .F. ) ;
#23085=CARTESIAN_POINT ( 'NONE',  ( 4.000000000000000888, 4.898587196589412829E-16, 16.50000000000001066 ) ) ;
#23086=CARTESIAN_POINT ( 'NONE',  ( 1.656854249492381470, 4.000000000000000000, 11.68750000000001066 ) ) ;
#23093=CARTESIAN_POINT ( 'NONE',  ( 2.445694354108822299, -2.445694354108820079, 19.06250000136560629 ) ) ;
#23105=CARTESIAN_POINT ( 'NONE',  ( -0.9413949561959078505, -0.3373062947069096484, -26.84672628368516811 ) ) ;
#23111=CARTESIAN_POINT ( 'NONE',  ( 3.458734125000001658, 4.235727675282972223E-16, 11.18750000136560452 ) ) ;
#23116=VECTOR ( 'NONE', #7289, 1000.000000000000000 ) ;
#23123=CARTESIAN_POINT ( 'NONE',  ( 4.000000000000000888, 4.898587196589412829E-16, 13.50000000000001066 ) ) ;
#23125=CARTESIAN_POINT ( 'NONE',  ( 1.432654583217643163, -3.458734124999999437, 16.75000000136560629 ) ) ;
#23128=EDGE_CURVE ( 'NONE', #4526, #17446, #6144, .T. ) ;
#23130=CARTESIAN_POINT ( 'NONE',  ( 4.000000000000000888, 4.898587196589412829E-16, 14.62500000273119660 ) ) ;
#23141=LINE ( 'NONE', #12044, #4482 ) ;
#23147=CARTESIAN_POINT ( 'NONE',  ( -1.432654583217639832, -3.458734125000000326, 15.87500000136560452 ) ) ;
#23171=DIRECTION ( 'NONE',  ( -0.000000000000000000, 1.000000000000000000, -0.000000000000000000 ) ) ;
#23172=UNCERTAINTY_MEASURE_WITH_UNIT (LENGTH_MEASURE( 1.000000000000000082E-05 ), #4493, 'distance_accuracy_value', 'NONE');
#23181=CARTESIAN_POINT ( 'NONE',  ( 1.432654583217641164, 3.458734125000000326, 13.12500000136560629 ) ) ;
#23199=DIRECTION ( 'NONE',  ( 0.000000000000000000, 0.000000000000000000, -1.000000000000000000 ) ) ;
#23207=CARTESIAN_POINT ( 'NONE',  ( 1.025207404391860050E-15, 3.458734125000000770, 19.43750000136560629 ) ) ;
#23222=EDGE_LOOP ( 'NONE', ( #115, #18004, #3385, #867 ) ) ;
#23228=CARTESIAN_POINT ( 'NONE',  ( -2.445694354108819191, 2.445694354108820523, 14.56250000136560452 ) ) ;
#23242=CARTESIAN_POINT ( 'NONE',  ( 3.458734125000001214, 4.235727675282971730E-16, 16.93750000136560629 ) ) ;
#23255=ORIENTED_EDGE ( 'NONE', *, *, #12450, .F. ) ;
#23256=CARTESIAN_POINT ( 'NONE',  ( -15.00000000000001066, 10.00000000000000000, -49.99999999999999289 ) ) ;
#23257=EDGE_CURVE ( 'NONE', #16922, #14633, #14178, .T. ) ;
#23259=ORIENTED_EDGE ( 'NONE', *, *, #10697, .T. ) ;
#23268=AXIS2_PLACEMENT_3D ( 'NONE', #8145, #19012, #19487 ) ;
#23271=CARTESIAN_POINT ( 'NONE',  ( 3.458734125000002546, -1.432654583217639610, 15.12500000136560807 ) ) ;
#23280=AXIS2_PLACEMENT_3D ( 'NONE', #7851, #9899, #4477 ) ;
#23281=ORIENTED_EDGE ( 'NONE', *, *, #784, .T. ) ;
#23290=LINE ( 'NONE', #18142, #19794 ) ;
#23291=AXIS2_PLACEMENT_3D ( 'NONE', #19231, #23171, #17686 ) ;
#23295=FACE_OUTER_BOUND ( 'NONE', #1418, .T. ) ;
#23297=CARTESIAN_POINT ( 'NONE',  ( 1.656854249492384135, -3.999999999999999112, 11.31250000000001066 ) ) ;
#23310=CARTESIAN_POINT ( 'NONE',  ( -3.999999999999999112, 0.000000000000000000, 13.12500000273119660 ) ) ;
#23311=CARTESIAN_POINT ( 'NONE',  ( -2.445694354108819191, 2.445694354108820523, 14.31250000136560452 ) ) ;
#23313=CARTESIAN_POINT ( 'NONE',  ( 1.236993788156008760E-15, 0.000000000000000000, 21.31370849898476649 ) ) ;
#23332=CARTESIAN_POINT ( 'NONE',  ( -3.999999999999999112, 0.000000000000000000, 16.00000000000001066 ) ) ;
#23335=ORIENTED_EDGE ( 'NONE', *, *, #12329, .T. ) ;
#23340=CARTESIAN_POINT ( 'NONE',  ( 2.445694354108821411, 2.445694354108820523, 18.31250000136560274 ) ) ;
#23343=CARTESIAN_POINT ( 'NONE',  ( -2.762848947613220307, 4.746226468750993632, 10.00000000000000888 ) ) ;
#23350=ORIENTED_EDGE ( 'NONE', *, *, #10697, .F. ) ;
#23360=CARTESIAN_POINT ( 'NONE',  ( 1.971781867644420635E-15, -4.000000000000000000, 17.25000000000001066 ) ) ;
#23364=CARTESIAN_POINT ( 'NONE',  ( 0.9413949561959078505, 0.3373062947069096484, -26.84672628368516811 ) ) ;
#23372=CARTESIAN_POINT ( 'NONE',  ( -1.432654583217639610, -3.458734124999999882, 18.62500000136560274 ) ) ;
#23383=ORIENTED_EDGE ( 'NONE', *, *, #22727, .T. ) ;
#23384=FACE_OUTER_BOUND ( 'NONE', #23222, .T. ) ;
#23385=EDGE_LOOP ( 'NONE', ( #4734, #7735, #5593, #14752 ) ) ;
#23392=CARTESIAN_POINT ( 'NONE',  ( -3.458734124999999437, 1.432654583217640498, 15.62500000136560629 ) ) ;
#23393=CARTESIAN_POINT ( 'NONE',  ( -2.828427124746189403, 2.828427124746190291, 10.00000000273119660 ) ) ;
#23412=CARTESIAN_POINT ( 'NONE',  ( -3.999999999999999112, 0.000000000000000000, 18.00000000000001066 ) ) ;
#23421=ADVANCED_FACE ( 'NONE', ( #20353 ), #3961, .T. ) ;
#23422=CIRCLE ( 'NONE', #15518, 4.000000000000000000 ) ;
#23425=PLANE ( 'NONE',  #17977 ) ;
#23429=CARTESIAN_POINT ( 'NONE',  ( 1.432654583217643163, -3.458734124999999437, 13.75000000136560452 ) ) ;
#23441=EDGE_LOOP ( 'NONE', ( #2819, #10994, #20267, #659 ) ) ;
#23460=FACE_OUTER_BOUND ( 'NONE', #9796, .T. ) ;
#23464=EDGE_CURVE ( 'NONE', #17728, #17488, #17026, .T. ) ;
#23469=PLANE ( 'NONE',  #16587 ) ;
#23474=CARTESIAN_POINT ( 'NONE',  ( -2.828427124746188515, -2.828427124746190735, 17.12500000000001066 ) ) ;
#23484=CARTESIAN_POINT ( 'NONE',  ( -2.247776618166700491, 3.308700692843503877, 10.00000000000000888 ) ) ;
#23486=CARTESIAN_POINT ( 'NONE',  ( -2.445694354108818303, -2.445694354108820523, 17.56250000136560274 ) ) ;
#23506=CARTESIAN_POINT ( 'NONE',  ( 1.872352939448454495E-15, -3.458734125000000770, 15.93750000136560629 ) ) ;
#23512=CARTESIAN_POINT ( 'NONE',  ( 2.828427124746192067, -2.828427124746189847, 18.50000000273119483 ) ) ;
#23526=CARTESIAN_POINT ( 'NONE',  ( -1.656854249492379250, 4.000000000000000000, 17.81250000000001421 ) ) ;
#23537=CARTESIAN_POINT ( 'NONE',  ( -3.999999999999999112, 0.000000000000000000, 14.00000000000001066 ) ) ;
#23542=CARTESIAN_POINT ( 'NONE',  ( -3.999999999999998224, -1.656854249492383024, 17.18750000273119838 ) ) ;
#23547=CARTESIAN_POINT ( 'NONE',  ( 1.432654583217643163, -3.458734124999999437, 16.75000000136560629 ) ) ;
#23564=CARTESIAN_POINT ( 'NONE',  ( -3.999999999999999112, 0.000000000000000000, 18.00000000000001066 ) ) ;
#23570=DIRECTION ( 'NONE',  ( 6.123233995736827666E-17, -1.000000000000000000, 0.000000000000000000 ) ) ;
#23573=ORIENTED_EDGE ( 'NONE', *, *, #7239, .F. ) ;
#23574=CARTESIAN_POINT ( 'NONE',  ( -3.999999999999999112, 0.000000000000000000, 18.12500000273119483 ) ) ;
#23583=CARTESIAN_POINT ( 'NONE',  ( 1.236993788156008760E-15, 0.000000000000000000, 21.31370849898476649 ) ) ;
#23585=CARTESIAN_POINT ( 'NONE',  ( -20.00000000000001066, 7.500000000000001776, -49.99999999999999289 ) ) ;
#23591=DIRECTION ( 'NONE',  ( -1.000000000000000000, 0.000000000000000000, 0.000000000000000000 ) ) ;
#23595=CARTESIAN_POINT ( 'NONE',  ( -3.999999999999999112, 1.656854249492380804, 16.93750000000001066 ) ) ;
#23596=DIRECTION ( 'NONE',  ( 0.000000000000000000, -1.000000000000000000, 0.000000000000000000 ) ) ;
#23605=CARTESIAN_POINT ( 'NONE',  ( -3.458734124999998993, 1.432654583217640276, 17.37500000136559919 ) ) ;
#23610=CARTESIAN_POINT ( 'NONE',  ( -1.432654583217638944, 3.458734125000000326, 19.25000000136560274 ) ) ;
#23624=CARTESIAN_POINT ( 'NONE',  ( -3.458734124999999437, 1.432654583217640498, 19.62500000136560629 ) ) ;
#23630=( BOUNDED_CURVE ( )  B_SPLINE_CURVE ( 2, ( #11943, #2685, #2795, #10025, #13495, #15295, #17312, #20647, #19208 ),
 .UNSPECIFIED., .F., .F. ) 
 B_SPLINE_CURVE_WITH_KNOTS ( ( 3, 2, 2, 2, 3 ),
 ( 0.4500000000000000111, 0.4625000000000000222, 0.4749999999999999778, 0.4874999999999999889, 0.5000000000000000000 ),
 .UNSPECIFIED. ) 
 CURVE ( )  GEOMETRIC_REPRESENTATION_ITEM ( )  RATIONAL_B_SPLINE_CURVE ( ( 1.000000000000000000, 0.9238795325112867385, 1.000000000000000000, 0.9238795325112867385, 1.000000000000000000, 0.9238795325112867385, 1.000000000000000000, 0.9238795325112867385, 1.000000000000000000 ) ) 
 REPRESENTATION_ITEM ( '' )  );
#23631=CARTESIAN_POINT ( 'NONE',  ( -3.458734124999999437, 0.000000000000000000, 16.68750000136560629 ) ) ;
#23632=CARTESIAN_POINT ( 'NONE',  ( 4.000000000000000888, 1.656854249492381248, 11.68750000273119660 ) ) ;
#23646=CYLINDRICAL_SURFACE ( 'NONE', #9388, 4.000000000000000000 ) ;
#23648=CARTESIAN_POINT ( 'NONE',  ( 4.000000000000001776, -1.656854249492379694, 18.43750000000000711 ) ) ;
#23660=DIRECTION ( 'NONE',  ( -0.000000000000000000, -0.000000000000000000, -1.000000000000000000 ) ) ;
#23670=CARTESIAN_POINT ( 'NONE',  ( 2.828427124746191179, 2.828427124746190291, 11.75000000273119660 ) ) ;
#23673=DIRECTION ( 'NONE',  ( 0.000000000000000000, 1.000000000000000000, 0.000000000000000000 ) ) ;
#23676=CARTESIAN_POINT ( 'NONE',  ( 4.000000000000000888, 1.656854249492381248, 13.68750000273119483 ) ) ;
#23684=VECTOR ( 'NONE', #3914, 1000.000000000000000 ) ;
#23692=CARTESIAN_POINT ( 'NONE',  ( 9.920644283265380691E-16, 4.000000000000000000, 16.87500000273119838 ) ) ;
ENDSEC;
END-ISO-10303-21;
